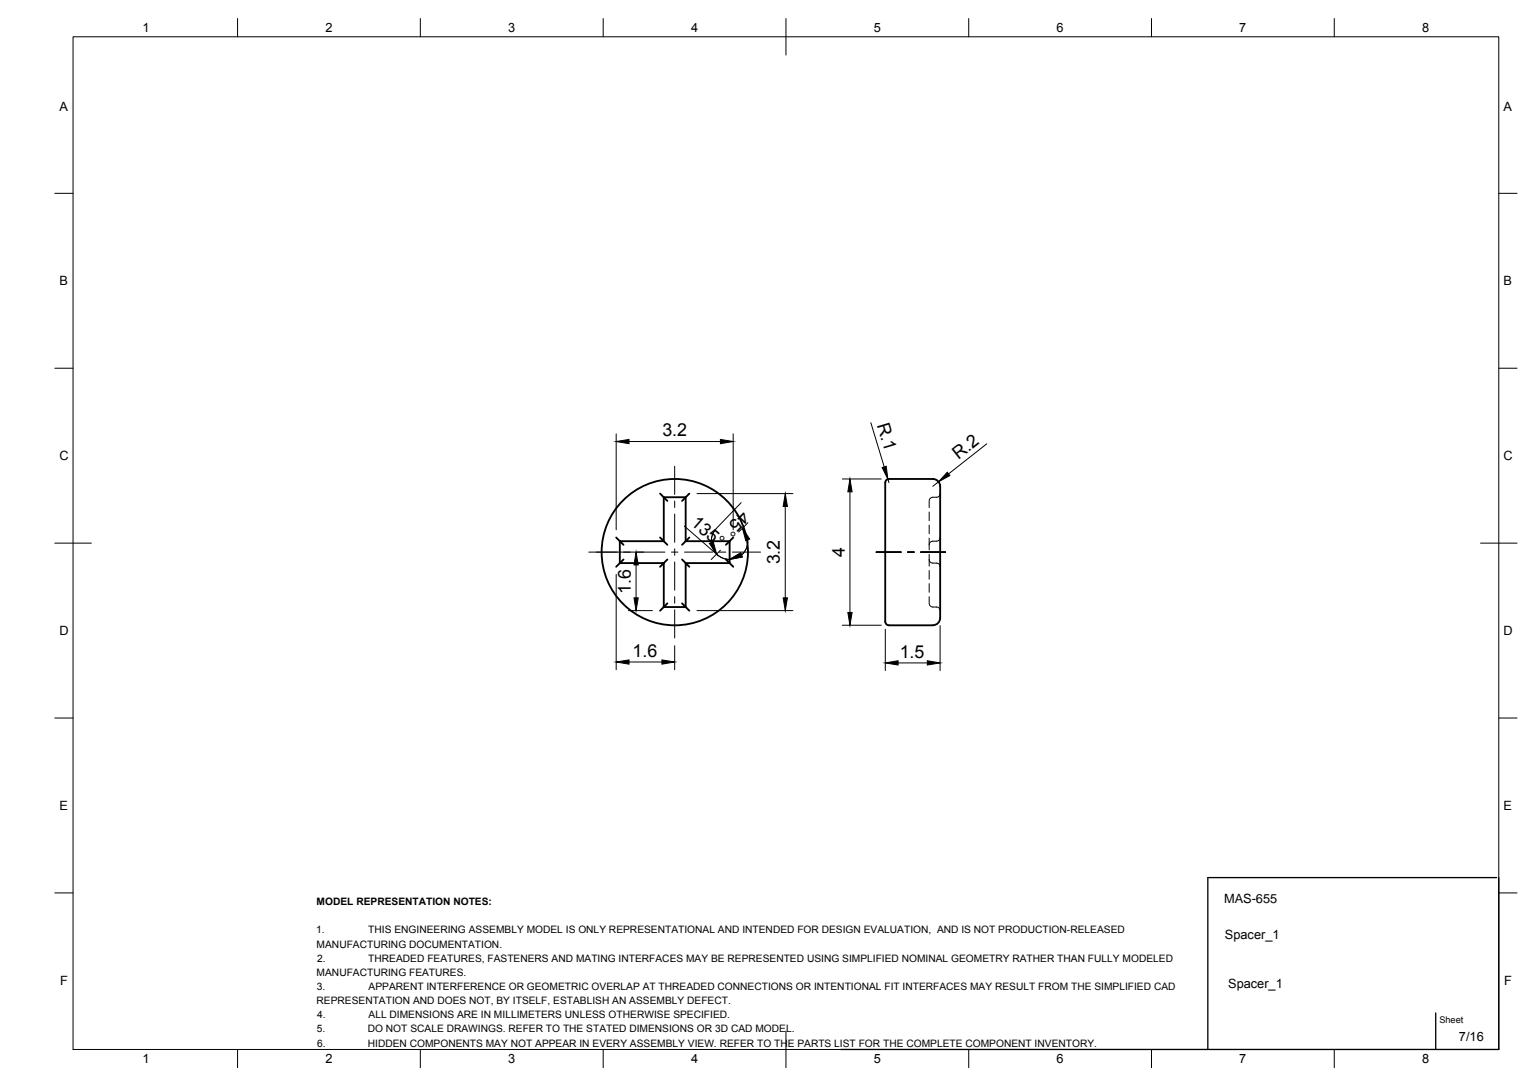
ISO-10303-21;
HEADER;
FILE_DESCRIPTION((''),'2;1');
FILE_NAME('Spacer_1.step','2026-10-09T11:34:15-07:00',(''),(''),'','','');
FILE_SCHEMA (('AUTOMOTIVE_DESIGN { 1 0 10303 214 3 1 1 }'));
ENDSEC;
DATA;
#10=MECHANICAL_DESIGN_GEOMETRIC_PRESENTATION_REPRESENTATION('',(#639),#117170);
#317=ELLIPSE('',#52230,0.141421356237297,0.1) ;
#318=ELLIPSE('',#52231,0.141421356237322,0.1) ;
#319=ELLIPSE('',#52233,0.141421356237322,0.1) ;
#320=ELLIPSE('',#52235,0.141421356237297,0.1) ;
#321=ELLIPSE('',#52237,0.141421356237322,0.1) ;
#322=ELLIPSE('',#52239,0.141421356237297,0.1) ;
#323=ELLIPSE('',#52241,0.141421356237297,0.1) ;
#324=ELLIPSE('',#52242,0.141421356237297,0.1) ;
#325=ELLIPSE('',#52244,0.141421356237322,0.1) ;
#326=ELLIPSE('',#52247,0.141421356237297,0.1) ;
#327=ELLIPSE('',#52249,0.141421356237322,0.1) ;
#328=ELLIPSE('',#52251,0.141421356237297,0.1) ;
#329=ELLIPSE('',#52262,0.141421356237272,0.1) ;
#330=ELLIPSE('',#52263,0.141421356237347,0.1) ;
#331=ELLIPSE('',#52265,0.141421356237347,0.1) ;
#332=ELLIPSE('',#52267,0.141421356237272,0.1) ;
#333=ELLIPSE('',#52269,0.141421356237297,0.1) ;
#334=ELLIPSE('',#52271,0.141421356237322,0.1) ;
#335=ELLIPSE('',#52273,0.141421356237347,0.1) ;
#336=ELLIPSE('',#52275,0.141421356237272,0.1) ;
#337=ELLIPSE('',#52277,0.141421356237347,0.1) ;
#338=ELLIPSE('',#52279,0.141421356237272,0.1) ;
#339=ELLIPSE('',#52281,0.141421356237297,0.1) ;
#340=ELLIPSE('',#52283,0.141421356237322,0.1) ;
#597=SHAPE_REPRESENTATION_RELATIONSHIP('SRR','None',#117252,#618) ;
#618=ADVANCED_BREP_SHAPE_REPRESENTATION('',(#660),#117160) ;
#639=STYLED_ITEM('',(#117355),#660) ;
#660=MANIFOLD_SOLID_BREP('Body1',#49068) ;
#734=FACE_BOUND('',#15393,.T.) ;
#2507=PLANE('',#52228) ;
#2508=PLANE('',#52253) ;
#2509=PLANE('',#52254) ;
#2510=PLANE('',#52255) ;
#2511=PLANE('',#52256) ;
#2512=PLANE('',#52257) ;
#2513=PLANE('',#52258) ;
#2514=PLANE('',#52259) ;
#2515=PLANE('',#52285) ;
#2516=PLANE('',#52286) ;
#2517=PLANE('',#52287) ;
#2518=PLANE('',#52288) ;
#2519=PLANE('',#52291) ;
#2520=PLANE('',#52292) ;
#2521=PLANE('',#52293) ;
#4366=LINE('',#88213,#7580) ;
#4367=LINE('',#88221,#7581) ;
#4368=LINE('',#88225,#7582) ;
#4369=LINE('',#88229,#7583) ;
#4370=LINE('',#88232,#7584) ;
#4371=LINE('',#88235,#7585) ;
#4372=LINE('',#88238,#7586) ;
#4373=LINE('',#88241,#7587) ;
#4374=LINE('',#88244,#7588) ;
#4375=LINE('',#88247,#7589) ;
#4376=LINE('',#88250,#7590) ;
#4377=LINE('',#88254,#7591) ;
#4378=LINE('',#88258,#7592) ;
#4379=LINE('',#88262,#7593) ;
#4380=LINE('',#88264,#7594) ;
#4381=LINE('',#88267,#7595) ;
#4382=LINE('',#88268,#7596) ;
#4383=LINE('',#88271,#7597) ;
#4384=LINE('',#88273,#7598) ;
#4385=LINE('',#88277,#7599) ;
#4386=LINE('',#88279,#7600) ;
#4387=LINE('',#88283,#7601) ;
#4388=LINE('',#88285,#7602) ;
#4389=LINE('',#88288,#7603) ;
#4390=LINE('',#88289,#7604) ;
#4391=LINE('',#88292,#7605) ;
#4392=LINE('',#88294,#7606) ;
#4393=LINE('',#88295,#7607) ;
#4394=LINE('',#88298,#7608) ;
#4395=LINE('',#88299,#7609) ;
#4396=LINE('',#88302,#7610) ;
#4397=LINE('',#88303,#7611) ;
#4398=LINE('',#88306,#7612) ;
#4399=LINE('',#88307,#7613) ;
#4400=LINE('',#88310,#7614) ;
#4401=LINE('',#88311,#7615) ;
#4402=LINE('',#88314,#7616) ;
#4403=LINE('',#88315,#7617) ;
#4404=LINE('',#88322,#7618) ;
#4405=LINE('',#88326,#7619) ;
#4406=LINE('',#88330,#7620) ;
#4407=LINE('',#88333,#7621) ;
#4408=LINE('',#88336,#7622) ;
#4409=LINE('',#88339,#7623) ;
#4410=LINE('',#88342,#7624) ;
#4411=LINE('',#88344,#7625) ;
#4412=LINE('',#88347,#7626) ;
#4413=LINE('',#88351,#7627) ;
#4414=LINE('',#88355,#7628) ;
#4415=LINE('',#88359,#7629) ;
#4416=LINE('',#88363,#7630) ;
#4417=LINE('',#88367,#7631) ;
#4418=LINE('',#88371,#7632) ;
#4419=LINE('',#88373,#7633) ;
#4420=LINE('',#88376,#7634) ;
#4421=LINE('',#88377,#7635) ;
#4422=LINE('',#88379,#7636) ;
#4423=LINE('',#88381,#7637) ;
#4424=LINE('',#88383,#7638) ;
#4425=LINE('',#88388,#7639) ;
#4426=LINE('',#88390,#7640) ;
#7580=VECTOR('',#62263,2.) ;
#7581=VECTOR('',#62272,10.) ;
#7582=VECTOR('',#62275,10.) ;
#7583=VECTOR('',#62280,10.) ;
#7584=VECTOR('',#62283,10.) ;
#7585=VECTOR('',#62286,10.) ;
#7586=VECTOR('',#62289,10.) ;
#7587=VECTOR('',#62292,10.) ;
#7588=VECTOR('',#62295,10.) ;
#7589=VECTOR('',#62298,10.) ;
#7590=VECTOR('',#62301,10.) ;
#7591=VECTOR('',#62304,10.) ;
#7592=VECTOR('',#62307,10.) ;
#7593=VECTOR('',#62312,10.) ;
#7594=VECTOR('',#62313,10.) ;
#7595=VECTOR('',#62318,10.) ;
#7596=VECTOR('',#62319,10.) ;
#7597=VECTOR('',#62322,10.) ;
#7598=VECTOR('',#62323,10.) ;
#7599=VECTOR('',#62328,10.) ;
#7600=VECTOR('',#62329,10.) ;
#7601=VECTOR('',#62334,10.) ;
#7602=VECTOR('',#62335,10.) ;
#7603=VECTOR('',#62340,10.) ;
#7604=VECTOR('',#62341,10.) ;
#7605=VECTOR('',#62344,10.) ;
#7606=VECTOR('',#62345,10.) ;
#7607=VECTOR('',#62346,10.) ;
#7608=VECTOR('',#62349,10.) ;
#7609=VECTOR('',#62350,10.) ;
#7610=VECTOR('',#62353,10.) ;
#7611=VECTOR('',#62354,10.) ;
#7612=VECTOR('',#62357,10.) ;
#7613=VECTOR('',#62358,10.) ;
#7614=VECTOR('',#62361,10.) ;
#7615=VECTOR('',#62362,10.) ;
#7616=VECTOR('',#62365,10.) ;
#7617=VECTOR('',#62366,10.) ;
#7618=VECTOR('',#62373,10.) ;
#7619=VECTOR('',#62376,10.) ;
#7620=VECTOR('',#62381,10.) ;
#7621=VECTOR('',#62384,10.) ;
#7622=VECTOR('',#62387,10.) ;
#7623=VECTOR('',#62390,10.) ;
#7624=VECTOR('',#62393,10.) ;
#7625=VECTOR('',#62396,10.) ;
#7626=VECTOR('',#62399,10.) ;
#7627=VECTOR('',#62404,10.) ;
#7628=VECTOR('',#62409,10.) ;
#7629=VECTOR('',#62414,10.) ;
#7630=VECTOR('',#62419,10.) ;
#7631=VECTOR('',#62424,10.) ;
#7632=VECTOR('',#62429,10.) ;
#7633=VECTOR('',#62430,10.) ;
#7634=VECTOR('',#62435,10.) ;
#7635=VECTOR('',#62436,10.) ;
#7636=VECTOR('',#62439,10.) ;
#7637=VECTOR('',#62442,10.) ;
#7638=VECTOR('',#62445,10.) ;
#7639=VECTOR('',#62454,10.) ;
#7640=VECTOR('',#62457,10.) ;
#10040=CYLINDRICAL_SURFACE('',#52225,2.) ;
#10041=CYLINDRICAL_SURFACE('',#52229,0.1) ;
#10042=CYLINDRICAL_SURFACE('',#52232,0.1) ;
#10043=CYLINDRICAL_SURFACE('',#52234,0.1) ;
#10044=CYLINDRICAL_SURFACE('',#52236,0.1) ;
#10045=CYLINDRICAL_SURFACE('',#52238,0.1) ;
#10046=CYLINDRICAL_SURFACE('',#52240,0.1) ;
#10047=CYLINDRICAL_SURFACE('',#52243,0.1) ;
#10048=CYLINDRICAL_SURFACE('',#52245,0.1) ;
#10049=CYLINDRICAL_SURFACE('',#52246,0.1) ;
#10050=CYLINDRICAL_SURFACE('',#52248,0.1) ;
#10051=CYLINDRICAL_SURFACE('',#52250,0.1) ;
#10052=CYLINDRICAL_SURFACE('',#52252,0.1) ;
#10053=CYLINDRICAL_SURFACE('',#52261,0.1) ;
#10054=CYLINDRICAL_SURFACE('',#52264,0.1) ;
#10055=CYLINDRICAL_SURFACE('',#52266,0.1) ;
#10056=CYLINDRICAL_SURFACE('',#52268,0.1) ;
#10057=CYLINDRICAL_SURFACE('',#52270,0.1) ;
#10058=CYLINDRICAL_SURFACE('',#52272,0.1) ;
#10059=CYLINDRICAL_SURFACE('',#52274,0.1) ;
#10060=CYLINDRICAL_SURFACE('',#52276,0.1) ;
#10061=CYLINDRICAL_SURFACE('',#52278,0.1) ;
#10062=CYLINDRICAL_SURFACE('',#52280,0.1) ;
#10063=CYLINDRICAL_SURFACE('',#52282,0.1) ;
#10064=CYLINDRICAL_SURFACE('',#52284,0.1) ;
#12215=FACE_OUTER_BOUND('',#15371,.T.) ;
#12216=FACE_OUTER_BOUND('',#15372,.T.) ;
#12217=FACE_OUTER_BOUND('',#15373,.T.) ;
#12218=FACE_OUTER_BOUND('',#15374,.T.) ;
#12219=FACE_OUTER_BOUND('',#15375,.T.) ;
#12220=FACE_OUTER_BOUND('',#15376,.T.) ;
#12221=FACE_OUTER_BOUND('',#15377,.T.) ;
#12222=FACE_OUTER_BOUND('',#15378,.T.) ;
#12223=FACE_OUTER_BOUND('',#15379,.T.) ;
#12224=FACE_OUTER_BOUND('',#15380,.T.) ;
#12225=FACE_OUTER_BOUND('',#15381,.T.) ;
#12226=FACE_OUTER_BOUND('',#15382,.T.) ;
#12227=FACE_OUTER_BOUND('',#15383,.T.) ;
#12228=FACE_OUTER_BOUND('',#15384,.T.) ;
#12229=FACE_OUTER_BOUND('',#15385,.T.) ;
#12230=FACE_OUTER_BOUND('',#15386,.T.) ;
#12231=FACE_OUTER_BOUND('',#15387,.T.) ;
#12232=FACE_OUTER_BOUND('',#15388,.T.) ;
#12233=FACE_OUTER_BOUND('',#15389,.T.) ;
#12234=FACE_OUTER_BOUND('',#15390,.T.) ;
#12235=FACE_OUTER_BOUND('',#15391,.T.) ;
#12236=FACE_OUTER_BOUND('',#15392,.T.) ;
#12237=FACE_OUTER_BOUND('',#15394,.T.) ;
#12238=FACE_OUTER_BOUND('',#15395,.T.) ;
#12239=FACE_OUTER_BOUND('',#15396,.T.) ;
#12240=FACE_OUTER_BOUND('',#15397,.T.) ;
#12241=FACE_OUTER_BOUND('',#15398,.T.) ;
#12242=FACE_OUTER_BOUND('',#15399,.T.) ;
#12243=FACE_OUTER_BOUND('',#15400,.T.) ;
#12244=FACE_OUTER_BOUND('',#15401,.T.) ;
#12245=FACE_OUTER_BOUND('',#15402,.T.) ;
#12246=FACE_OUTER_BOUND('',#15403,.T.) ;
#12247=FACE_OUTER_BOUND('',#15404,.T.) ;
#12248=FACE_OUTER_BOUND('',#15405,.T.) ;
#12249=FACE_OUTER_BOUND('',#15406,.T.) ;
#12250=FACE_OUTER_BOUND('',#15407,.T.) ;
#12251=FACE_OUTER_BOUND('',#15408,.T.) ;
#12252=FACE_OUTER_BOUND('',#15409,.T.) ;
#12253=FACE_OUTER_BOUND('',#15410,.T.) ;
#12254=FACE_OUTER_BOUND('',#15411,.T.) ;
#12255=FACE_OUTER_BOUND('',#15412,.T.) ;
#12256=FACE_OUTER_BOUND('',#15413,.T.) ;
#15371=EDGE_LOOP('',(#37742,#37743,#37744,#37745,#37746)) ;
#15372=EDGE_LOOP('',(#37747,#37748,#37749,#37750,#37751,#37752)) ;
#15373=EDGE_LOOP('',(#37753)) ;
#15374=EDGE_LOOP('',(#37754,#37755,#37756,#37757)) ;
#15375=EDGE_LOOP('',(#37758,#37759,#37760,#37761)) ;
#15376=EDGE_LOOP('',(#37762,#37763,#37764,#37765)) ;
#15377=EDGE_LOOP('',(#37766,#37767,#37768,#37769)) ;
#15378=EDGE_LOOP('',(#37770,#37771,#37772,#37773)) ;
#15379=EDGE_LOOP('',(#37774,#37775,#37776,#37777)) ;
#15380=EDGE_LOOP('',(#37778,#37779,#37780,#37781)) ;
#15381=EDGE_LOOP('',(#37782,#37783,#37784,#37785)) ;
#15382=EDGE_LOOP('',(#37786,#37787,#37788,#37789)) ;
#15383=EDGE_LOOP('',(#37790,#37791,#37792,#37793)) ;
#15384=EDGE_LOOP('',(#37794,#37795,#37796,#37797)) ;
#15385=EDGE_LOOP('',(#37798,#37799,#37800,#37801)) ;
#15386=EDGE_LOOP('',(#37802,#37803,#37804,#37805)) ;
#15387=EDGE_LOOP('',(#37806,#37807,#37808,#37809)) ;
#15388=EDGE_LOOP('',(#37810,#37811,#37812,#37813)) ;
#15389=EDGE_LOOP('',(#37814,#37815,#37816,#37817)) ;
#15390=EDGE_LOOP('',(#37818,#37819,#37820,#37821)) ;
#15391=EDGE_LOOP('',(#37822,#37823,#37824,#37825)) ;
#15392=EDGE_LOOP('',(#37826)) ;
#15393=EDGE_LOOP('',(#37827,#37828,#37829,#37830,#37831,#37832,#37833,#37834,
#37835,#37836,#37837,#37838)) ;
#15394=EDGE_LOOP('',(#37839,#37840,#37841,#37842)) ;
#15395=EDGE_LOOP('',(#37843,#37844,#37845,#37846)) ;
#15396=EDGE_LOOP('',(#37847,#37848,#37849,#37850)) ;
#15397=EDGE_LOOP('',(#37851,#37852,#37853,#37854)) ;
#15398=EDGE_LOOP('',(#37855,#37856,#37857,#37858)) ;
#15399=EDGE_LOOP('',(#37859,#37860,#37861,#37862)) ;
#15400=EDGE_LOOP('',(#37863,#37864,#37865,#37866)) ;
#15401=EDGE_LOOP('',(#37867,#37868,#37869,#37870)) ;
#15402=EDGE_LOOP('',(#37871,#37872,#37873,#37874)) ;
#15403=EDGE_LOOP('',(#37875,#37876,#37877,#37878)) ;
#15404=EDGE_LOOP('',(#37879,#37880,#37881,#37882)) ;
#15405=EDGE_LOOP('',(#37883,#37884,#37885,#37886)) ;
#15406=EDGE_LOOP('',(#37887,#37888,#37889,#37890)) ;
#15407=EDGE_LOOP('',(#37891,#37892,#37893,#37894)) ;
#15408=EDGE_LOOP('',(#37895,#37896,#37897,#37898)) ;
#15409=EDGE_LOOP('',(#37899,#37900,#37901,#37902,#37903,#37904,#37905,#37906,
#37907,#37908,#37909,#37910)) ;
#15410=EDGE_LOOP('',(#37911,#37912,#37913,#37914,#37915)) ;
#15411=EDGE_LOOP('',(#37916,#37917,#37918,#37919)) ;
#15412=EDGE_LOOP('',(#37920,#37921,#37922,#37923)) ;
#15413=EDGE_LOOP('',(#37924,#37925,#37926,#37927)) ;
#18485=CIRCLE('',#52221,1.9) ;
#18486=CIRCLE('',#52222,0.1) ;
#18487=CIRCLE('',#52223,2.) ;
#18488=CIRCLE('',#52224,2.) ;
#18489=CIRCLE('',#52226,2.) ;
#18490=CIRCLE('',#52227,2.) ;
#18491=CIRCLE('',#52260,1.8) ;
#18492=CIRCLE('',#52290,0.2) ;
#21507=VERTEX_POINT('',#88204) ;
#21508=VERTEX_POINT('',#88206) ;
#21509=VERTEX_POINT('',#88208) ;
#21510=VERTEX_POINT('',#88212) ;
#21511=VERTEX_POINT('',#88214) ;
#21512=VERTEX_POINT('',#88219) ;
#21513=VERTEX_POINT('',#88220) ;
#21514=VERTEX_POINT('',#88222) ;
#21515=VERTEX_POINT('',#88224) ;
#21516=VERTEX_POINT('',#88228) ;
#21517=VERTEX_POINT('',#88230) ;
#21518=VERTEX_POINT('',#88234) ;
#21519=VERTEX_POINT('',#88236) ;
#21520=VERTEX_POINT('',#88240) ;
#21521=VERTEX_POINT('',#88242) ;
#21522=VERTEX_POINT('',#88246) ;
#21523=VERTEX_POINT('',#88248) ;
#21524=VERTEX_POINT('',#88252) ;
#21525=VERTEX_POINT('',#88253) ;
#21526=VERTEX_POINT('',#88255) ;
#21527=VERTEX_POINT('',#88257) ;
#21528=VERTEX_POINT('',#88261) ;
#21529=VERTEX_POINT('',#88263) ;
#21530=VERTEX_POINT('',#88270) ;
#21531=VERTEX_POINT('',#88272) ;
#21532=VERTEX_POINT('',#88276) ;
#21533=VERTEX_POINT('',#88278) ;
#21534=VERTEX_POINT('',#88282) ;
#21535=VERTEX_POINT('',#88284) ;
#21536=VERTEX_POINT('',#88291) ;
#21537=VERTEX_POINT('',#88293) ;
#21538=VERTEX_POINT('',#88297) ;
#21539=VERTEX_POINT('',#88301) ;
#21540=VERTEX_POINT('',#88305) ;
#21541=VERTEX_POINT('',#88309) ;
#21542=VERTEX_POINT('',#88313) ;
#21543=VERTEX_POINT('',#88317) ;
#21544=VERTEX_POINT('',#88320) ;
#21545=VERTEX_POINT('',#88321) ;
#21546=VERTEX_POINT('',#88323) ;
#21547=VERTEX_POINT('',#88325) ;
#21548=VERTEX_POINT('',#88329) ;
#21549=VERTEX_POINT('',#88331) ;
#21550=VERTEX_POINT('',#88335) ;
#21551=VERTEX_POINT('',#88337) ;
#21552=VERTEX_POINT('',#88341) ;
#21553=VERTEX_POINT('',#88346) ;
#21554=VERTEX_POINT('',#88350) ;
#21555=VERTEX_POINT('',#88354) ;
#21556=VERTEX_POINT('',#88358) ;
#21557=VERTEX_POINT('',#88362) ;
#21558=VERTEX_POINT('',#88366) ;
#21559=VERTEX_POINT('',#88370) ;
#21560=VERTEX_POINT('',#88372) ;
#27149=EDGE_CURVE('',#21507,#21507,#18485,.T.) ;
#27150=EDGE_CURVE('',#21507,#21508,#18486,.T.) ;
#27151=EDGE_CURVE('',#21508,#21509,#18487,.T.) ;
#27152=EDGE_CURVE('',#21509,#21508,#18488,.T.) ;
#27153=EDGE_CURVE('',#21509,#21510,#4366,.T.) ;
#27154=EDGE_CURVE('',#21511,#21510,#18489,.T.) ;
#27155=EDGE_CURVE('',#21510,#21511,#18490,.T.) ;
#27156=EDGE_CURVE('',#21512,#21513,#4367,.T.) ;
#27157=EDGE_CURVE('',#21513,#21514,#317,.T.) ;
#27158=EDGE_CURVE('',#21514,#21515,#4368,.T.) ;
#27159=EDGE_CURVE('',#21512,#21515,#318,.T.) ;
#27160=EDGE_CURVE('',#21513,#21516,#4369,.T.) ;
#27161=EDGE_CURVE('',#21516,#21517,#319,.T.) ;
#27162=EDGE_CURVE('',#21517,#21514,#4370,.T.) ;
#27163=EDGE_CURVE('',#21516,#21518,#4371,.T.) ;
#27164=EDGE_CURVE('',#21518,#21519,#320,.T.) ;
#27165=EDGE_CURVE('',#21519,#21517,#4372,.T.) ;
#27166=EDGE_CURVE('',#21518,#21520,#4373,.T.) ;
#27167=EDGE_CURVE('',#21520,#21521,#321,.T.) ;
#27168=EDGE_CURVE('',#21521,#21519,#4374,.T.) ;
#27169=EDGE_CURVE('',#21520,#21522,#4375,.T.) ;
#27170=EDGE_CURVE('',#21522,#21523,#322,.T.) ;
#27171=EDGE_CURVE('',#21523,#21521,#4376,.T.) ;
#27172=EDGE_CURVE('',#21524,#21525,#4377,.T.) ;
#27173=EDGE_CURVE('',#21525,#21526,#323,.T.) ;
#27174=EDGE_CURVE('',#21526,#21527,#4378,.T.) ;
#27175=EDGE_CURVE('',#21527,#21524,#324,.T.) ;
#27176=EDGE_CURVE('',#21528,#21526,#4379,.T.) ;
#27177=EDGE_CURVE('',#21525,#21529,#4380,.T.) ;
#27178=EDGE_CURVE('',#21529,#21528,#325,.T.) ;
#27179=EDGE_CURVE('',#21522,#21524,#4381,.T.) ;
#27180=EDGE_CURVE('',#21527,#21523,#4382,.T.) ;
#27181=EDGE_CURVE('',#21530,#21528,#4383,.T.) ;
#27182=EDGE_CURVE('',#21529,#21531,#4384,.T.) ;
#27183=EDGE_CURVE('',#21531,#21530,#326,.T.) ;
#27184=EDGE_CURVE('',#21532,#21530,#4385,.T.) ;
#27185=EDGE_CURVE('',#21531,#21533,#4386,.T.) ;
#27186=EDGE_CURVE('',#21533,#21532,#327,.T.) ;
#27187=EDGE_CURVE('',#21534,#21532,#4387,.T.) ;
#27188=EDGE_CURVE('',#21533,#21535,#4388,.T.) ;
#27189=EDGE_CURVE('',#21535,#21534,#328,.T.) ;
#27190=EDGE_CURVE('',#21515,#21534,#4389,.T.) ;
#27191=EDGE_CURVE('',#21535,#21512,#4390,.T.) ;
#27192=EDGE_CURVE('',#21517,#21536,#4391,.T.) ;
#27193=EDGE_CURVE('',#21537,#21536,#4392,.T.) ;
#27194=EDGE_CURVE('',#21514,#21537,#4393,.T.) ;
#27195=EDGE_CURVE('',#21519,#21538,#4394,.T.) ;
#27196=EDGE_CURVE('',#21536,#21538,#4395,.T.) ;
#27197=EDGE_CURVE('',#21521,#21539,#4396,.T.) ;
#27198=EDGE_CURVE('',#21538,#21539,#4397,.T.) ;
#27199=EDGE_CURVE('',#21523,#21540,#4398,.T.) ;
#27200=EDGE_CURVE('',#21539,#21540,#4399,.T.) ;
#27201=EDGE_CURVE('',#21527,#21541,#4400,.T.) ;
#27202=EDGE_CURVE('',#21540,#21541,#4401,.T.) ;
#27203=EDGE_CURVE('',#21526,#21542,#4402,.T.) ;
#27204=EDGE_CURVE('',#21541,#21542,#4403,.T.) ;
#27205=EDGE_CURVE('',#21543,#21543,#18491,.T.) ;
#27206=EDGE_CURVE('',#21544,#21545,#4404,.T.) ;
#27207=EDGE_CURVE('',#21545,#21546,#329,.T.) ;
#27208=EDGE_CURVE('',#21546,#21547,#4405,.T.) ;
#27209=EDGE_CURVE('',#21544,#21547,#330,.T.) ;
#27210=EDGE_CURVE('',#21545,#21548,#4406,.T.) ;
#27211=EDGE_CURVE('',#21548,#21549,#331,.T.) ;
#27212=EDGE_CURVE('',#21549,#21546,#4407,.T.) ;
#27213=EDGE_CURVE('',#21548,#21550,#4408,.T.) ;
#27214=EDGE_CURVE('',#21550,#21551,#332,.T.) ;
#27215=EDGE_CURVE('',#21551,#21549,#4409,.T.) ;
#27216=EDGE_CURVE('',#21550,#21552,#4410,.T.) ;
#27217=EDGE_CURVE('',#21552,#21542,#333,.T.) ;
#27218=EDGE_CURVE('',#21542,#21551,#4411,.T.) ;
#27219=EDGE_CURVE('',#21552,#21553,#4412,.T.) ;
#27220=EDGE_CURVE('',#21553,#21541,#334,.T.) ;
#27221=EDGE_CURVE('',#21553,#21554,#4413,.T.) ;
#27222=EDGE_CURVE('',#21554,#21540,#335,.T.) ;
#27223=EDGE_CURVE('',#21554,#21555,#4414,.T.) ;
#27224=EDGE_CURVE('',#21555,#21539,#336,.T.) ;
#27225=EDGE_CURVE('',#21555,#21556,#4415,.T.) ;
#27226=EDGE_CURVE('',#21556,#21538,#337,.T.) ;
#27227=EDGE_CURVE('',#21556,#21557,#4416,.T.) ;
#27228=EDGE_CURVE('',#21557,#21536,#338,.T.) ;
#27229=EDGE_CURVE('',#21557,#21558,#4417,.T.) ;
#27230=EDGE_CURVE('',#21558,#21537,#339,.T.) ;
#27231=EDGE_CURVE('',#21559,#21537,#4418,.T.) ;
#27232=EDGE_CURVE('',#21558,#21560,#4419,.T.) ;
#27233=EDGE_CURVE('',#21560,#21559,#340,.T.) ;
#27234=EDGE_CURVE('',#21547,#21559,#4420,.T.) ;
#27235=EDGE_CURVE('',#21560,#21544,#4421,.T.) ;
#27236=EDGE_CURVE('',#21515,#21559,#4422,.T.) ;
#27237=EDGE_CURVE('',#21534,#21547,#4423,.T.) ;
#27238=EDGE_CURVE('',#21532,#21546,#4424,.T.) ;
#27239=EDGE_CURVE('',#21511,#21543,#18492,.T.) ;
#27240=EDGE_CURVE('',#21530,#21549,#4425,.T.) ;
#27241=EDGE_CURVE('',#21528,#21551,#4426,.T.) ;
#37742=ORIENTED_EDGE('',*,*,#27149,.T.) ;
#37743=ORIENTED_EDGE('',*,*,#27150,.T.) ;
#37744=ORIENTED_EDGE('',*,*,#27151,.T.) ;
#37745=ORIENTED_EDGE('',*,*,#27152,.T.) ;
#37746=ORIENTED_EDGE('',*,*,#27150,.F.) ;
#37747=ORIENTED_EDGE('',*,*,#27152,.F.) ;
#37748=ORIENTED_EDGE('',*,*,#27153,.T.) ;
#37749=ORIENTED_EDGE('',*,*,#27154,.F.) ;
#37750=ORIENTED_EDGE('',*,*,#27155,.F.) ;
#37751=ORIENTED_EDGE('',*,*,#27153,.F.) ;
#37752=ORIENTED_EDGE('',*,*,#27151,.F.) ;
#37753=ORIENTED_EDGE('',*,*,#27149,.F.) ;
#37754=ORIENTED_EDGE('',*,*,#27156,.T.) ;
#37755=ORIENTED_EDGE('',*,*,#27157,.T.) ;
#37756=ORIENTED_EDGE('',*,*,#27158,.T.) ;
#37757=ORIENTED_EDGE('',*,*,#27159,.F.) ;
#37758=ORIENTED_EDGE('',*,*,#27160,.T.) ;
#37759=ORIENTED_EDGE('',*,*,#27161,.T.) ;
#37760=ORIENTED_EDGE('',*,*,#27162,.T.) ;
#37761=ORIENTED_EDGE('',*,*,#27157,.F.) ;
#37762=ORIENTED_EDGE('',*,*,#27163,.T.) ;
#37763=ORIENTED_EDGE('',*,*,#27164,.T.) ;
#37764=ORIENTED_EDGE('',*,*,#27165,.T.) ;
#37765=ORIENTED_EDGE('',*,*,#27161,.F.) ;
#37766=ORIENTED_EDGE('',*,*,#27166,.T.) ;
#37767=ORIENTED_EDGE('',*,*,#27167,.T.) ;
#37768=ORIENTED_EDGE('',*,*,#27168,.T.) ;
#37769=ORIENTED_EDGE('',*,*,#27164,.F.) ;
#37770=ORIENTED_EDGE('',*,*,#27169,.T.) ;
#37771=ORIENTED_EDGE('',*,*,#27170,.T.) ;
#37772=ORIENTED_EDGE('',*,*,#27171,.T.) ;
#37773=ORIENTED_EDGE('',*,*,#27167,.F.) ;
#37774=ORIENTED_EDGE('',*,*,#27172,.T.) ;
#37775=ORIENTED_EDGE('',*,*,#27173,.T.) ;
#37776=ORIENTED_EDGE('',*,*,#27174,.T.) ;
#37777=ORIENTED_EDGE('',*,*,#27175,.T.) ;
#37778=ORIENTED_EDGE('',*,*,#27176,.T.) ;
#37779=ORIENTED_EDGE('',*,*,#27173,.F.) ;
#37780=ORIENTED_EDGE('',*,*,#27177,.T.) ;
#37781=ORIENTED_EDGE('',*,*,#27178,.T.) ;
#37782=ORIENTED_EDGE('',*,*,#27179,.T.) ;
#37783=ORIENTED_EDGE('',*,*,#27175,.F.) ;
#37784=ORIENTED_EDGE('',*,*,#27180,.T.) ;
#37785=ORIENTED_EDGE('',*,*,#27170,.F.) ;
#37786=ORIENTED_EDGE('',*,*,#27181,.T.) ;
#37787=ORIENTED_EDGE('',*,*,#27178,.F.) ;
#37788=ORIENTED_EDGE('',*,*,#27182,.T.) ;
#37789=ORIENTED_EDGE('',*,*,#27183,.T.) ;
#37790=ORIENTED_EDGE('',*,*,#27184,.T.) ;
#37791=ORIENTED_EDGE('',*,*,#27183,.F.) ;
#37792=ORIENTED_EDGE('',*,*,#27185,.T.) ;
#37793=ORIENTED_EDGE('',*,*,#27186,.T.) ;
#37794=ORIENTED_EDGE('',*,*,#27187,.T.) ;
#37795=ORIENTED_EDGE('',*,*,#27186,.F.) ;
#37796=ORIENTED_EDGE('',*,*,#27188,.T.) ;
#37797=ORIENTED_EDGE('',*,*,#27189,.T.) ;
#37798=ORIENTED_EDGE('',*,*,#27190,.T.) ;
#37799=ORIENTED_EDGE('',*,*,#27189,.F.) ;
#37800=ORIENTED_EDGE('',*,*,#27191,.T.) ;
#37801=ORIENTED_EDGE('',*,*,#27159,.T.) ;
#37802=ORIENTED_EDGE('',*,*,#27162,.F.) ;
#37803=ORIENTED_EDGE('',*,*,#27192,.T.) ;
#37804=ORIENTED_EDGE('',*,*,#27193,.F.) ;
#37805=ORIENTED_EDGE('',*,*,#27194,.F.) ;
#37806=ORIENTED_EDGE('',*,*,#27165,.F.) ;
#37807=ORIENTED_EDGE('',*,*,#27195,.T.) ;
#37808=ORIENTED_EDGE('',*,*,#27196,.F.) ;
#37809=ORIENTED_EDGE('',*,*,#27192,.F.) ;
#37810=ORIENTED_EDGE('',*,*,#27168,.F.) ;
#37811=ORIENTED_EDGE('',*,*,#27197,.T.) ;
#37812=ORIENTED_EDGE('',*,*,#27198,.F.) ;
#37813=ORIENTED_EDGE('',*,*,#27195,.F.) ;
#37814=ORIENTED_EDGE('',*,*,#27171,.F.) ;
#37815=ORIENTED_EDGE('',*,*,#27199,.T.) ;
#37816=ORIENTED_EDGE('',*,*,#27200,.F.) ;
#37817=ORIENTED_EDGE('',*,*,#27197,.F.) ;
#37818=ORIENTED_EDGE('',*,*,#27180,.F.) ;
#37819=ORIENTED_EDGE('',*,*,#27201,.T.) ;
#37820=ORIENTED_EDGE('',*,*,#27202,.F.) ;
#37821=ORIENTED_EDGE('',*,*,#27199,.F.) ;
#37822=ORIENTED_EDGE('',*,*,#27174,.F.) ;
#37823=ORIENTED_EDGE('',*,*,#27203,.T.) ;
#37824=ORIENTED_EDGE('',*,*,#27204,.F.) ;
#37825=ORIENTED_EDGE('',*,*,#27201,.F.) ;
#37826=ORIENTED_EDGE('',*,*,#27205,.F.) ;
#37827=ORIENTED_EDGE('',*,*,#27172,.F.) ;
#37828=ORIENTED_EDGE('',*,*,#27179,.F.) ;
#37829=ORIENTED_EDGE('',*,*,#27169,.F.) ;
#37830=ORIENTED_EDGE('',*,*,#27166,.F.) ;
#37831=ORIENTED_EDGE('',*,*,#27163,.F.) ;
#37832=ORIENTED_EDGE('',*,*,#27160,.F.) ;
#37833=ORIENTED_EDGE('',*,*,#27156,.F.) ;
#37834=ORIENTED_EDGE('',*,*,#27191,.F.) ;
#37835=ORIENTED_EDGE('',*,*,#27188,.F.) ;
#37836=ORIENTED_EDGE('',*,*,#27185,.F.) ;
#37837=ORIENTED_EDGE('',*,*,#27182,.F.) ;
#37838=ORIENTED_EDGE('',*,*,#27177,.F.) ;
#37839=ORIENTED_EDGE('',*,*,#27206,.T.) ;
#37840=ORIENTED_EDGE('',*,*,#27207,.T.) ;
#37841=ORIENTED_EDGE('',*,*,#27208,.T.) ;
#37842=ORIENTED_EDGE('',*,*,#27209,.F.) ;
#37843=ORIENTED_EDGE('',*,*,#27210,.T.) ;
#37844=ORIENTED_EDGE('',*,*,#27211,.T.) ;
#37845=ORIENTED_EDGE('',*,*,#27212,.T.) ;
#37846=ORIENTED_EDGE('',*,*,#27207,.F.) ;
#37847=ORIENTED_EDGE('',*,*,#27213,.T.) ;
#37848=ORIENTED_EDGE('',*,*,#27214,.T.) ;
#37849=ORIENTED_EDGE('',*,*,#27215,.T.) ;
#37850=ORIENTED_EDGE('',*,*,#27211,.F.) ;
#37851=ORIENTED_EDGE('',*,*,#27216,.T.) ;
#37852=ORIENTED_EDGE('',*,*,#27217,.T.) ;
#37853=ORIENTED_EDGE('',*,*,#27218,.T.) ;
#37854=ORIENTED_EDGE('',*,*,#27214,.F.) ;
#37855=ORIENTED_EDGE('',*,*,#27219,.T.) ;
#37856=ORIENTED_EDGE('',*,*,#27220,.T.) ;
#37857=ORIENTED_EDGE('',*,*,#27204,.T.) ;
#37858=ORIENTED_EDGE('',*,*,#27217,.F.) ;
#37859=ORIENTED_EDGE('',*,*,#27202,.T.) ;
#37860=ORIENTED_EDGE('',*,*,#27220,.F.) ;
#37861=ORIENTED_EDGE('',*,*,#27221,.T.) ;
#37862=ORIENTED_EDGE('',*,*,#27222,.T.) ;
#37863=ORIENTED_EDGE('',*,*,#27200,.T.) ;
#37864=ORIENTED_EDGE('',*,*,#27222,.F.) ;
#37865=ORIENTED_EDGE('',*,*,#27223,.T.) ;
#37866=ORIENTED_EDGE('',*,*,#27224,.T.) ;
#37867=ORIENTED_EDGE('',*,*,#27198,.T.) ;
#37868=ORIENTED_EDGE('',*,*,#27224,.F.) ;
#37869=ORIENTED_EDGE('',*,*,#27225,.T.) ;
#37870=ORIENTED_EDGE('',*,*,#27226,.T.) ;
#37871=ORIENTED_EDGE('',*,*,#27196,.T.) ;
#37872=ORIENTED_EDGE('',*,*,#27226,.F.) ;
#37873=ORIENTED_EDGE('',*,*,#27227,.T.) ;
#37874=ORIENTED_EDGE('',*,*,#27228,.T.) ;
#37875=ORIENTED_EDGE('',*,*,#27193,.T.) ;
#37876=ORIENTED_EDGE('',*,*,#27228,.F.) ;
#37877=ORIENTED_EDGE('',*,*,#27229,.T.) ;
#37878=ORIENTED_EDGE('',*,*,#27230,.T.) ;
#37879=ORIENTED_EDGE('',*,*,#27231,.T.) ;
#37880=ORIENTED_EDGE('',*,*,#27230,.F.) ;
#37881=ORIENTED_EDGE('',*,*,#27232,.T.) ;
#37882=ORIENTED_EDGE('',*,*,#27233,.T.) ;
#37883=ORIENTED_EDGE('',*,*,#27234,.T.) ;
#37884=ORIENTED_EDGE('',*,*,#27233,.F.) ;
#37885=ORIENTED_EDGE('',*,*,#27235,.T.) ;
#37886=ORIENTED_EDGE('',*,*,#27209,.T.) ;
#37887=ORIENTED_EDGE('',*,*,#27158,.F.) ;
#37888=ORIENTED_EDGE('',*,*,#27194,.T.) ;
#37889=ORIENTED_EDGE('',*,*,#27231,.F.) ;
#37890=ORIENTED_EDGE('',*,*,#27236,.F.) ;
#37891=ORIENTED_EDGE('',*,*,#27190,.F.) ;
#37892=ORIENTED_EDGE('',*,*,#27236,.T.) ;
#37893=ORIENTED_EDGE('',*,*,#27234,.F.) ;
#37894=ORIENTED_EDGE('',*,*,#27237,.F.) ;
#37895=ORIENTED_EDGE('',*,*,#27187,.F.) ;
#37896=ORIENTED_EDGE('',*,*,#27237,.T.) ;
#37897=ORIENTED_EDGE('',*,*,#27208,.F.) ;
#37898=ORIENTED_EDGE('',*,*,#27238,.F.) ;
#37899=ORIENTED_EDGE('',*,*,#27206,.F.) ;
#37900=ORIENTED_EDGE('',*,*,#27235,.F.) ;
#37901=ORIENTED_EDGE('',*,*,#27232,.F.) ;
#37902=ORIENTED_EDGE('',*,*,#27229,.F.) ;
#37903=ORIENTED_EDGE('',*,*,#27227,.F.) ;
#37904=ORIENTED_EDGE('',*,*,#27225,.F.) ;
#37905=ORIENTED_EDGE('',*,*,#27223,.F.) ;
#37906=ORIENTED_EDGE('',*,*,#27221,.F.) ;
#37907=ORIENTED_EDGE('',*,*,#27219,.F.) ;
#37908=ORIENTED_EDGE('',*,*,#27216,.F.) ;
#37909=ORIENTED_EDGE('',*,*,#27213,.F.) ;
#37910=ORIENTED_EDGE('',*,*,#27210,.F.) ;
#37911=ORIENTED_EDGE('',*,*,#27154,.T.) ;
#37912=ORIENTED_EDGE('',*,*,#27155,.T.) ;
#37913=ORIENTED_EDGE('',*,*,#27239,.T.) ;
#37914=ORIENTED_EDGE('',*,*,#27205,.T.) ;
#37915=ORIENTED_EDGE('',*,*,#27239,.F.) ;
#37916=ORIENTED_EDGE('',*,*,#27184,.F.) ;
#37917=ORIENTED_EDGE('',*,*,#27238,.T.) ;
#37918=ORIENTED_EDGE('',*,*,#27212,.F.) ;
#37919=ORIENTED_EDGE('',*,*,#27240,.F.) ;
#37920=ORIENTED_EDGE('',*,*,#27181,.F.) ;
#37921=ORIENTED_EDGE('',*,*,#27240,.T.) ;
#37922=ORIENTED_EDGE('',*,*,#27215,.F.) ;
#37923=ORIENTED_EDGE('',*,*,#27241,.F.) ;
#37924=ORIENTED_EDGE('',*,*,#27176,.F.) ;
#37925=ORIENTED_EDGE('',*,*,#27241,.T.) ;
#37926=ORIENTED_EDGE('',*,*,#27218,.F.) ;
#37927=ORIENTED_EDGE('',*,*,#27203,.F.) ;
#45707=TOROIDAL_SURFACE('',#52220,1.9,0.1) ;
#45708=TOROIDAL_SURFACE('',#52289,1.8,0.2) ;
#47433=ADVANCED_FACE('',(#12215),#45707,.T.) ;
#47434=ADVANCED_FACE('',(#12216),#10040,.T.) ;
#47435=ADVANCED_FACE('',(#12217),#2507,.T.) ;
#47436=ADVANCED_FACE('',(#12218),#10041,.T.) ;
#47437=ADVANCED_FACE('',(#12219),#10042,.T.) ;
#47438=ADVANCED_FACE('',(#12220),#10043,.T.) ;
#47439=ADVANCED_FACE('',(#12221),#10044,.T.) ;
#47440=ADVANCED_FACE('',(#12222),#10045,.T.) ;
#47441=ADVANCED_FACE('',(#12223),#10046,.T.) ;
#47442=ADVANCED_FACE('',(#12224),#10047,.T.) ;
#47443=ADVANCED_FACE('',(#12225),#10048,.T.) ;
#47444=ADVANCED_FACE('',(#12226),#10049,.T.) ;
#47445=ADVANCED_FACE('',(#12227),#10050,.T.) ;
#47446=ADVANCED_FACE('',(#12228),#10051,.T.) ;
#47447=ADVANCED_FACE('',(#12229),#10052,.T.) ;
#47448=ADVANCED_FACE('',(#12230),#2508,.F.) ;
#47449=ADVANCED_FACE('',(#12231),#2509,.F.) ;
#47450=ADVANCED_FACE('',(#12232),#2510,.F.) ;
#47451=ADVANCED_FACE('',(#12233),#2511,.F.) ;
#47452=ADVANCED_FACE('',(#12234),#2512,.F.) ;
#47453=ADVANCED_FACE('',(#12235),#2513,.F.) ;
#47454=ADVANCED_FACE('',(#12236,#734),#2514,.F.) ;
#47455=ADVANCED_FACE('',(#12237),#10053,.F.) ;
#47456=ADVANCED_FACE('',(#12238),#10054,.F.) ;
#47457=ADVANCED_FACE('',(#12239),#10055,.F.) ;
#47458=ADVANCED_FACE('',(#12240),#10056,.F.) ;
#47459=ADVANCED_FACE('',(#12241),#10057,.F.) ;
#47460=ADVANCED_FACE('',(#12242),#10058,.F.) ;
#47461=ADVANCED_FACE('',(#12243),#10059,.F.) ;
#47462=ADVANCED_FACE('',(#12244),#10060,.F.) ;
#47463=ADVANCED_FACE('',(#12245),#10061,.F.) ;
#47464=ADVANCED_FACE('',(#12246),#10062,.F.) ;
#47465=ADVANCED_FACE('',(#12247),#10063,.F.) ;
#47466=ADVANCED_FACE('',(#12248),#10064,.F.) ;
#47467=ADVANCED_FACE('',(#12249),#2515,.F.) ;
#47468=ADVANCED_FACE('',(#12250),#2516,.F.) ;
#47469=ADVANCED_FACE('',(#12251),#2517,.F.) ;
#47470=ADVANCED_FACE('',(#12252),#2518,.F.) ;
#47471=ADVANCED_FACE('',(#12253),#45708,.T.) ;
#47472=ADVANCED_FACE('',(#12254),#2519,.F.) ;
#47473=ADVANCED_FACE('',(#12255),#2520,.F.) ;
#47474=ADVANCED_FACE('',(#12256),#2521,.F.) ;
#49068=CLOSED_SHELL('',(#47433,#47434,#47435,#47436,#47437,#47438,#47439,
#47440,#47441,#47442,#47443,#47444,#47445,#47446,#47447,#47448,#47449,#47450,
#47451,#47452,#47453,#47454,#47455,#47456,#47457,#47458,#47459,#47460,#47461,
#47462,#47463,#47464,#47465,#47466,#47467,#47468,#47469,#47470,#47471,#47472,
#47473,#47474)) ;
#52219=AXIS2_PLACEMENT_3D('',#88202,#62249,#62250) ;
#52220=AXIS2_PLACEMENT_3D('',#88203,#62251,#62252) ;
#52221=AXIS2_PLACEMENT_3D('',#88205,#62253,#62254) ;
#52222=AXIS2_PLACEMENT_3D('',#88207,#62255,#62256) ;
#52223=AXIS2_PLACEMENT_3D('',#88209,#62257,#62258) ;
#52224=AXIS2_PLACEMENT_3D('',#88210,#62259,#62260) ;
#52225=AXIS2_PLACEMENT_3D('',#88211,#62261,#62262) ;
#52226=AXIS2_PLACEMENT_3D('',#88215,#62264,#62265) ;
#52227=AXIS2_PLACEMENT_3D('',#88216,#62266,#62267) ;
#52228=AXIS2_PLACEMENT_3D('',#88217,#62268,#62269) ;
#52229=AXIS2_PLACEMENT_3D('',#88218,#62270,#62271) ;
#52230=AXIS2_PLACEMENT_3D('',#88223,#62273,#62274) ;
#52231=AXIS2_PLACEMENT_3D('',#88226,#62276,#62277) ;
#52232=AXIS2_PLACEMENT_3D('',#88227,#62278,#62279) ;
#52233=AXIS2_PLACEMENT_3D('',#88231,#62281,#62282) ;
#52234=AXIS2_PLACEMENT_3D('',#88233,#62284,#62285) ;
#52235=AXIS2_PLACEMENT_3D('',#88237,#62287,#62288) ;
#52236=AXIS2_PLACEMENT_3D('',#88239,#62290,#62291) ;
#52237=AXIS2_PLACEMENT_3D('',#88243,#62293,#62294) ;
#52238=AXIS2_PLACEMENT_3D('',#88245,#62296,#62297) ;
#52239=AXIS2_PLACEMENT_3D('',#88249,#62299,#62300) ;
#52240=AXIS2_PLACEMENT_3D('',#88251,#62302,#62303) ;
#52241=AXIS2_PLACEMENT_3D('',#88256,#62305,#62306) ;
#52242=AXIS2_PLACEMENT_3D('',#88259,#62308,#62309) ;
#52243=AXIS2_PLACEMENT_3D('',#88260,#62310,#62311) ;
#52244=AXIS2_PLACEMENT_3D('',#88265,#62314,#62315) ;
#52245=AXIS2_PLACEMENT_3D('',#88266,#62316,#62317) ;
#52246=AXIS2_PLACEMENT_3D('',#88269,#62320,#62321) ;
#52247=AXIS2_PLACEMENT_3D('',#88274,#62324,#62325) ;
#52248=AXIS2_PLACEMENT_3D('',#88275,#62326,#62327) ;
#52249=AXIS2_PLACEMENT_3D('',#88280,#62330,#62331) ;
#52250=AXIS2_PLACEMENT_3D('',#88281,#62332,#62333) ;
#52251=AXIS2_PLACEMENT_3D('',#88286,#62336,#62337) ;
#52252=AXIS2_PLACEMENT_3D('',#88287,#62338,#62339) ;
#52253=AXIS2_PLACEMENT_3D('',#88290,#62342,#62343) ;
#52254=AXIS2_PLACEMENT_3D('',#88296,#62347,#62348) ;
#52255=AXIS2_PLACEMENT_3D('',#88300,#62351,#62352) ;
#52256=AXIS2_PLACEMENT_3D('',#88304,#62355,#62356) ;
#52257=AXIS2_PLACEMENT_3D('',#88308,#62359,#62360) ;
#52258=AXIS2_PLACEMENT_3D('',#88312,#62363,#62364) ;
#52259=AXIS2_PLACEMENT_3D('',#88316,#62367,#62368) ;
#52260=AXIS2_PLACEMENT_3D('',#88318,#62369,#62370) ;
#52261=AXIS2_PLACEMENT_3D('',#88319,#62371,#62372) ;
#52262=AXIS2_PLACEMENT_3D('',#88324,#62374,#62375) ;
#52263=AXIS2_PLACEMENT_3D('',#88327,#62377,#62378) ;
#52264=AXIS2_PLACEMENT_3D('',#88328,#62379,#62380) ;
#52265=AXIS2_PLACEMENT_3D('',#88332,#62382,#62383) ;
#52266=AXIS2_PLACEMENT_3D('',#88334,#62385,#62386) ;
#52267=AXIS2_PLACEMENT_3D('',#88338,#62388,#62389) ;
#52268=AXIS2_PLACEMENT_3D('',#88340,#62391,#62392) ;
#52269=AXIS2_PLACEMENT_3D('',#88343,#62394,#62395) ;
#52270=AXIS2_PLACEMENT_3D('',#88345,#62397,#62398) ;
#52271=AXIS2_PLACEMENT_3D('',#88348,#62400,#62401) ;
#52272=AXIS2_PLACEMENT_3D('',#88349,#62402,#62403) ;
#52273=AXIS2_PLACEMENT_3D('',#88352,#62405,#62406) ;
#52274=AXIS2_PLACEMENT_3D('',#88353,#62407,#62408) ;
#52275=AXIS2_PLACEMENT_3D('',#88356,#62410,#62411) ;
#52276=AXIS2_PLACEMENT_3D('',#88357,#62412,#62413) ;
#52277=AXIS2_PLACEMENT_3D('',#88360,#62415,#62416) ;
#52278=AXIS2_PLACEMENT_3D('',#88361,#62417,#62418) ;
#52279=AXIS2_PLACEMENT_3D('',#88364,#62420,#62421) ;
#52280=AXIS2_PLACEMENT_3D('',#88365,#62422,#62423) ;
#52281=AXIS2_PLACEMENT_3D('',#88368,#62425,#62426) ;
#52282=AXIS2_PLACEMENT_3D('',#88369,#62427,#62428) ;
#52283=AXIS2_PLACEMENT_3D('',#88374,#62431,#62432) ;
#52284=AXIS2_PLACEMENT_3D('',#88375,#62433,#62434) ;
#52285=AXIS2_PLACEMENT_3D('',#88378,#62437,#62438) ;
#52286=AXIS2_PLACEMENT_3D('',#88380,#62440,#62441) ;
#52287=AXIS2_PLACEMENT_3D('',#88382,#62443,#62444) ;
#52288=AXIS2_PLACEMENT_3D('',#88384,#62446,#62447) ;
#52289=AXIS2_PLACEMENT_3D('',#88385,#62448,#62449) ;
#52290=AXIS2_PLACEMENT_3D('',#88386,#62450,#62451) ;
#52291=AXIS2_PLACEMENT_3D('',#88387,#62452,#62453) ;
#52292=AXIS2_PLACEMENT_3D('',#88389,#62455,#62456) ;
#52293=AXIS2_PLACEMENT_3D('',#88391,#62458,#62459) ;
#62249=DIRECTION('axis',(0.,0.,1.)) ;
#62250=DIRECTION('refdir',(1.,0.,0.)) ;
#62251=DIRECTION('center_axis',(2.52374105052742E-18,5.60383084497445E-34,
-1.)) ;
#62252=DIRECTION('ref_axis',(-1.,0.,0.)) ;
#62253=DIRECTION('center_axis',(-2.52374105052742E-18,-5.60383084497445E-34,
1.)) ;
#62254=DIRECTION('ref_axis',(1.,-2.80191542248716E-35,2.52374105052742E-18)) ;
#62255=DIRECTION('center_axis',(0.,-1.,-5.60383084497445E-34)) ;
#62256=DIRECTION('ref_axis',(1.,0.,0.)) ;
#62257=DIRECTION('center_axis',(2.52374105052742E-18,5.60383084497445E-34,
-1.)) ;
#62258=DIRECTION('ref_axis',(1.,-2.80191542248716E-35,2.52374105052742E-18)) ;
#62259=DIRECTION('center_axis',(2.52374105052742E-18,5.60383084497445E-34,
-1.)) ;
#62260=DIRECTION('ref_axis',(1.,-2.80191542248716E-35,2.52374105052742E-18)) ;
#62261=DIRECTION('center_axis',(0.,0.,-1.)) ;
#62262=DIRECTION('ref_axis',(1.,0.,0.)) ;
#62263=DIRECTION('',(0.,0.,1.)) ;
#62264=DIRECTION('center_axis',(-2.52374105052742E-18,-5.60383084497445E-34,
1.)) ;
#62265=DIRECTION('ref_axis',(1.,5.60383084497445E-35,2.52374105052742E-18)) ;
#62266=DIRECTION('center_axis',(-2.52374105052742E-18,-5.60383084497445E-34,
1.)) ;
#62267=DIRECTION('ref_axis',(1.,5.60383084497445E-35,2.52374105052742E-18)) ;
#62268=DIRECTION('center_axis',(2.52374105052742E-18,5.60383084497445E-34,
-1.)) ;
#62269=DIRECTION('ref_axis',(1.,3.40207761657885E-68,2.52374105052742E-18)) ;
#62270=DIRECTION('center_axis',(-1.,0.,-2.52374105052742E-18)) ;
#62271=DIRECTION('ref_axis',(-1.78455441078696E-18,0.707106781186485,0.70710678118661)) ;
#62272=DIRECTION('',(1.,0.,2.52374105052742E-18)) ;
#62273=DIRECTION('center_axis',(-0.70710678118661,-0.707106781186485,0.)) ;
#62274=DIRECTION('ref_axis',(0.707106781186485,-0.70710678118661,3.56910882157392E-18)) ;
#62275=DIRECTION('',(-1.,0.,-2.52374105052742E-18)) ;
#62276=DIRECTION('center_axis',(-0.70710678118661,0.707106781186485,0.)) ;
#62277=DIRECTION('ref_axis',(-0.707106781186485,-0.70710678118661,-7.92501358220685E-34)) ;
#62278=DIRECTION('center_axis',(1.41426179436738E-51,-1.,-5.60383084497445E-34)) ;
#62279=DIRECTION('ref_axis',(-0.707106781186548,-3.96250679110377E-34,0.707106781186548)) ;
#62280=DIRECTION('',(-1.41426179436738E-51,1.,5.60383084497445E-34)) ;
#62281=DIRECTION('center_axis',(-0.70710678118661,-0.707106781186485,0.)) ;
#62282=DIRECTION('ref_axis',(-0.707106781186485,0.70710678118661,7.92501358220685E-34)) ;
#62283=DIRECTION('',(1.41426179436738E-51,-1.,-5.60383084497445E-34)) ;
#62284=DIRECTION('center_axis',(-1.,0.,-2.52374105052742E-18)) ;
#62285=DIRECTION('ref_axis',(-1.78455441078696E-18,0.707106781186485,0.70710678118661)) ;
#62286=DIRECTION('',(1.,0.,2.52374105052742E-18)) ;
#62287=DIRECTION('center_axis',(-0.70710678118661,-0.707106781186485,0.)) ;
#62288=DIRECTION('ref_axis',(0.707106781186485,-0.70710678118661,3.56910882157392E-18)) ;
#62289=DIRECTION('',(-1.,0.,-2.52374105052742E-18)) ;
#62290=DIRECTION('center_axis',(1.41426179436738E-51,-1.,-5.60383084497445E-34)) ;
#62291=DIRECTION('ref_axis',(-0.707106781186548,-3.96250679110377E-34,0.707106781186548)) ;
#62292=DIRECTION('',(-1.41426179436738E-51,1.,5.60383084497445E-34)) ;
#62293=DIRECTION('center_axis',(0.70710678118661,-0.707106781186485,0.)) ;
#62294=DIRECTION('ref_axis',(0.707106781186485,0.70710678118661,7.92501358220685E-34)) ;
#62295=DIRECTION('',(1.41426179436738E-51,-1.,-5.60383084497445E-34)) ;
#62296=DIRECTION('center_axis',(1.,0.,2.52374105052742E-18)) ;
#62297=DIRECTION('ref_axis',(-1.78455441078696E-18,-0.707106781186485,0.70710678118661)) ;
#62298=DIRECTION('',(-1.,0.,-2.52374105052742E-18)) ;
#62299=DIRECTION('center_axis',(0.70710678118661,-0.707106781186485,0.)) ;
#62300=DIRECTION('ref_axis',(-0.707106781186485,-0.70710678118661,-3.56910882157392E-18)) ;
#62301=DIRECTION('',(1.,0.,2.52374105052742E-18)) ;
#62302=DIRECTION('center_axis',(1.,0.,2.52374105052742E-18)) ;
#62303=DIRECTION('ref_axis',(-1.78455441078696E-18,-0.707106781186485,0.70710678118661)) ;
#62304=DIRECTION('',(-1.,0.,-2.52374105052742E-18)) ;
#62305=DIRECTION('center_axis',(0.70710678118661,0.707106781186485,0.)) ;
#62306=DIRECTION('ref_axis',(-0.707106781186485,0.70710678118661,-3.56910882157392E-18)) ;
#62307=DIRECTION('',(1.,0.,2.52374105052742E-18)) ;
#62308=DIRECTION('center_axis',(-0.70710678118661,0.707106781186485,0.)) ;
#62309=DIRECTION('ref_axis',(-0.707106781186485,-0.70710678118661,-3.56910882157392E-18)) ;
#62310=DIRECTION('center_axis',(-1.41426179436738E-51,1.,5.60383084497445E-34)) ;
#62311=DIRECTION('ref_axis',(0.707106781186548,-3.96250679110377E-34,0.707106781186548)) ;
#62312=DIRECTION('',(-1.41426179436738E-51,1.,5.60383084497445E-34)) ;
#62313=DIRECTION('',(1.41426179436738E-51,-1.,-5.60383084497445E-34)) ;
#62314=DIRECTION('center_axis',(0.70710678118661,0.707106781186485,0.)) ;
#62315=DIRECTION('ref_axis',(0.707106781186485,-0.70710678118661,-7.92501358220685E-34)) ;
#62316=DIRECTION('center_axis',(1.41426179436738E-51,-1.,-5.60383084497445E-34)) ;
#62317=DIRECTION('ref_axis',(-0.707106781186548,-3.96250679110377E-34,0.707106781186548)) ;
#62318=DIRECTION('',(-1.41426179436738E-51,1.,5.60383084497445E-34)) ;
#62319=DIRECTION('',(1.41426179436738E-51,-1.,-5.60383084497445E-34)) ;
#62320=DIRECTION('center_axis',(1.,0.,2.52374105052742E-18)) ;
#62321=DIRECTION('ref_axis',(-1.78455441078696E-18,-0.707106781186485,0.70710678118661)) ;
#62322=DIRECTION('',(1.,0.,2.52374105052742E-18)) ;
#62323=DIRECTION('',(-1.,0.,-2.52374105052742E-18)) ;
#62324=DIRECTION('center_axis',(0.70710678118661,0.707106781186485,0.)) ;
#62325=DIRECTION('ref_axis',(-0.707106781186485,0.70710678118661,-3.56910882157392E-18)) ;
#62326=DIRECTION('center_axis',(-1.41426179436738E-51,1.,5.60383084497445E-34)) ;
#62327=DIRECTION('ref_axis',(0.707106781186548,-3.96250679110377E-34,0.707106781186548)) ;
#62328=DIRECTION('',(-1.41426179436738E-51,1.,5.60383084497445E-34)) ;
#62329=DIRECTION('',(1.41426179436738E-51,-1.,-5.60383084497445E-34)) ;
#62330=DIRECTION('center_axis',(-0.70710678118661,0.707106781186485,0.)) ;
#62331=DIRECTION('ref_axis',(-0.707106781186485,-0.70710678118661,-7.92501358220685E-34)) ;
#62332=DIRECTION('center_axis',(-1.,0.,-2.52374105052742E-18)) ;
#62333=DIRECTION('ref_axis',(-1.78455441078696E-18,0.707106781186485,0.70710678118661)) ;
#62334=DIRECTION('',(-1.,0.,-2.52374105052742E-18)) ;
#62335=DIRECTION('',(1.,0.,2.52374105052742E-18)) ;
#62336=DIRECTION('center_axis',(-0.70710678118661,0.707106781186485,0.)) ;
#62337=DIRECTION('ref_axis',(0.707106781186485,0.70710678118661,3.56910882157392E-18)) ;
#62338=DIRECTION('center_axis',(-1.41426179436738E-51,1.,5.60383084497445E-34)) ;
#62339=DIRECTION('ref_axis',(0.707106781186548,-3.96250679110377E-34,0.707106781186548)) ;
#62340=DIRECTION('',(-1.41426179436738E-51,1.,5.60383084497445E-34)) ;
#62341=DIRECTION('',(1.41426179436738E-51,-1.,-5.60383084497445E-34)) ;
#62342=DIRECTION('center_axis',(1.,1.41426179436738E-51,0.)) ;
#62343=DIRECTION('ref_axis',(1.41426179436738E-51,-1.,-5.60383084497445E-34)) ;
#62344=DIRECTION('',(0.,0.,-1.)) ;
#62345=DIRECTION('',(-1.41426179436738E-51,1.,0.)) ;
#62346=DIRECTION('',(0.,0.,-1.)) ;
#62347=DIRECTION('center_axis',(0.,-1.,0.)) ;
#62348=DIRECTION('ref_axis',(-1.,0.,-2.52374105052742E-18)) ;
#62349=DIRECTION('',(0.,0.,-1.)) ;
#62350=DIRECTION('',(1.,0.,0.)) ;
#62351=DIRECTION('center_axis',(1.,1.41426179436738E-51,0.)) ;
#62352=DIRECTION('ref_axis',(1.41426179436738E-51,-1.,-5.60383084497445E-34)) ;
#62353=DIRECTION('',(0.,0.,-1.)) ;
#62354=DIRECTION('',(-1.41426179436738E-51,1.,0.)) ;
#62355=DIRECTION('center_axis',(0.,1.,0.)) ;
#62356=DIRECTION('ref_axis',(1.,0.,2.52374105052742E-18)) ;
#62357=DIRECTION('',(0.,0.,-1.)) ;
#62358=DIRECTION('',(-1.,0.,0.)) ;
#62359=DIRECTION('center_axis',(1.,1.41426179436738E-51,0.)) ;
#62360=DIRECTION('ref_axis',(1.41426179436738E-51,-1.,-5.60383084497445E-34)) ;
#62361=DIRECTION('',(0.,0.,-1.)) ;
#62362=DIRECTION('',(-1.41426179436738E-51,1.,0.)) ;
#62363=DIRECTION('center_axis',(0.,1.,0.)) ;
#62364=DIRECTION('ref_axis',(1.,0.,2.52374105052742E-18)) ;
#62365=DIRECTION('',(0.,0.,-1.)) ;
#62366=DIRECTION('',(-1.,0.,0.)) ;
#62367=DIRECTION('center_axis',(2.52374105052742E-18,5.60383084497445E-34,
-1.)) ;
#62368=DIRECTION('ref_axis',(1.,3.40207761657885E-68,2.52374105052742E-18)) ;
#62369=DIRECTION('center_axis',(2.52374105052742E-18,5.60383084497445E-34,
-1.)) ;
#62370=DIRECTION('ref_axis',(1.,5.60383084497445E-35,2.52374105052742E-18)) ;
#62371=DIRECTION('center_axis',(-1.,0.,0.)) ;
#62372=DIRECTION('ref_axis',(0.,-0.707106781186736,-0.707106781186359)) ;
#62373=DIRECTION('',(-1.,0.,0.)) ;
#62374=DIRECTION('center_axis',(-0.707106781186736,0.707106781186359,0.)) ;
#62375=DIRECTION('ref_axis',(0.707106781186359,0.707106781186736,0.)) ;
#62376=DIRECTION('',(1.,0.,0.)) ;
#62377=DIRECTION('center_axis',(-0.707106781186736,0.707106781186359,0.)) ;
#62378=DIRECTION('ref_axis',(-0.707106781186359,-0.707106781186736,0.)) ;
#62379=DIRECTION('center_axis',(-1.41426179436738E-51,1.,0.)) ;
#62380=DIRECTION('ref_axis',(-0.707106781186548,-1.00003410517023E-51,-0.707106781186548)) ;
#62381=DIRECTION('',(-1.41426179436738E-51,1.,0.)) ;
#62382=DIRECTION('center_axis',(0.707106781186736,0.707106781186359,0.)) ;
#62383=DIRECTION('ref_axis',(0.707106781186359,-0.707106781186736,0.)) ;
#62384=DIRECTION('',(1.41426179436738E-51,-1.,0.)) ;
#62385=DIRECTION('center_axis',(1.,0.,0.)) ;
#62386=DIRECTION('ref_axis',(0.,0.707106781186736,-0.707106781186359)) ;
#62387=DIRECTION('',(1.,0.,0.)) ;
#62388=DIRECTION('center_axis',(0.707106781186736,0.707106781186359,0.)) ;
#62389=DIRECTION('ref_axis',(-0.707106781186359,0.707106781186736,0.)) ;
#62390=DIRECTION('',(-1.,0.,0.)) ;
#62391=DIRECTION('center_axis',(-1.41426179436738E-51,1.,0.)) ;
#62392=DIRECTION('ref_axis',(-0.707106781186548,-1.00003410517023E-51,-0.707106781186548)) ;
#62393=DIRECTION('',(-1.41426179436738E-51,1.,0.)) ;
#62394=DIRECTION('center_axis',(0.707106781186485,0.70710678118661,0.)) ;
#62395=DIRECTION('ref_axis',(0.70710678118661,-0.707106781186485,0.)) ;
#62396=DIRECTION('',(1.41426179436738E-51,-1.,0.)) ;
#62397=DIRECTION('center_axis',(1.,0.,0.)) ;
#62398=DIRECTION('ref_axis',(0.,0.707106781186485,-0.70710678118661)) ;
#62399=DIRECTION('',(1.,0.,0.)) ;
#62400=DIRECTION('center_axis',(0.707106781186485,-0.70710678118661,0.)) ;
#62401=DIRECTION('ref_axis',(-0.70710678118661,-0.707106781186485,0.)) ;
#62402=DIRECTION('center_axis',(1.41426179436738E-51,-1.,0.)) ;
#62403=DIRECTION('ref_axis',(0.707106781186548,1.00003410517023E-51,-0.707106781186548)) ;
#62404=DIRECTION('',(1.41426179436738E-51,-1.,0.)) ;
#62405=DIRECTION('center_axis',(0.707106781186736,-0.707106781186359,0.)) ;
#62406=DIRECTION('ref_axis',(0.707106781186359,0.707106781186736,0.)) ;
#62407=DIRECTION('center_axis',(1.,0.,0.)) ;
#62408=DIRECTION('ref_axis',(0.,0.707106781186736,-0.707106781186359)) ;
#62409=DIRECTION('',(1.,0.,0.)) ;
#62410=DIRECTION('center_axis',(0.707106781186736,-0.707106781186359,0.)) ;
#62411=DIRECTION('ref_axis',(-0.707106781186359,-0.707106781186736,0.)) ;
#62412=DIRECTION('center_axis',(1.41426179436738E-51,-1.,0.)) ;
#62413=DIRECTION('ref_axis',(0.707106781186548,1.00003410517023E-51,-0.707106781186548)) ;
#62414=DIRECTION('',(1.41426179436738E-51,-1.,0.)) ;
#62415=DIRECTION('center_axis',(-0.707106781186736,-0.707106781186359,0.)) ;
#62416=DIRECTION('ref_axis',(-0.707106781186359,0.707106781186736,0.)) ;
#62417=DIRECTION('center_axis',(-1.,0.,0.)) ;
#62418=DIRECTION('ref_axis',(0.,-0.707106781186736,-0.707106781186359)) ;
#62419=DIRECTION('',(-1.,0.,0.)) ;
#62420=DIRECTION('center_axis',(-0.707106781186736,-0.707106781186359,0.)) ;
#62421=DIRECTION('ref_axis',(0.707106781186359,-0.707106781186736,0.)) ;
#62422=DIRECTION('center_axis',(1.41426179436738E-51,-1.,0.)) ;
#62423=DIRECTION('ref_axis',(0.707106781186548,1.00003410517023E-51,-0.707106781186548)) ;
#62424=DIRECTION('',(1.41426179436738E-51,-1.,0.)) ;
#62425=DIRECTION('center_axis',(-0.707106781186485,-0.70710678118661,0.)) ;
#62426=DIRECTION('ref_axis',(-0.70710678118661,0.707106781186485,0.)) ;
#62427=DIRECTION('center_axis',(-1.,0.,0.)) ;
#62428=DIRECTION('ref_axis',(0.,-0.707106781186485,-0.70710678118661)) ;
#62429=DIRECTION('',(1.,0.,0.)) ;
#62430=DIRECTION('',(-1.,0.,0.)) ;
#62431=DIRECTION('center_axis',(-0.707106781186485,0.70710678118661,0.)) ;
#62432=DIRECTION('ref_axis',(0.70710678118661,0.707106781186485,0.)) ;
#62433=DIRECTION('center_axis',(-1.41426179436738E-51,1.,0.)) ;
#62434=DIRECTION('ref_axis',(-0.707106781186548,-1.00003410517023E-51,-0.707106781186548)) ;
#62435=DIRECTION('',(1.41426179436738E-51,-1.,0.)) ;
#62436=DIRECTION('',(-1.41426179436738E-51,1.,0.)) ;
#62437=DIRECTION('center_axis',(0.,-1.,0.)) ;
#62438=DIRECTION('ref_axis',(-1.,0.,-2.52374105052742E-18)) ;
#62439=DIRECTION('',(0.,0.,-1.)) ;
#62440=DIRECTION('center_axis',(-1.,-1.41426179436738E-51,0.)) ;
#62441=DIRECTION('ref_axis',(-1.41426179436738E-51,1.,5.60383084497445E-34)) ;
#62442=DIRECTION('',(0.,0.,-1.)) ;
#62443=DIRECTION('center_axis',(0.,-1.,0.)) ;
#62444=DIRECTION('ref_axis',(-1.,0.,-2.52374105052742E-18)) ;
#62445=DIRECTION('',(0.,0.,-1.)) ;
#62446=DIRECTION('center_axis',(0.,0.,-1.)) ;
#62447=DIRECTION('ref_axis',(-1.,0.,0.)) ;
#62448=DIRECTION('center_axis',(2.52374105052742E-18,5.60383084497445E-34,
-1.)) ;
#62449=DIRECTION('ref_axis',(-1.,0.,0.)) ;
#62450=DIRECTION('center_axis',(0.,-1.,-5.60383084497445E-34)) ;
#62451=DIRECTION('ref_axis',(1.,0.,0.)) ;
#62452=DIRECTION('center_axis',(-1.,-1.41426179436738E-51,0.)) ;
#62453=DIRECTION('ref_axis',(-1.41426179436738E-51,1.,5.60383084497445E-34)) ;
#62454=DIRECTION('',(0.,0.,-1.)) ;
#62455=DIRECTION('center_axis',(0.,1.,0.)) ;
#62456=DIRECTION('ref_axis',(1.,0.,2.52374105052742E-18)) ;
#62457=DIRECTION('',(0.,0.,-1.)) ;
#62458=DIRECTION('center_axis',(-1.,-1.41426179436738E-51,0.)) ;
#62459=DIRECTION('ref_axis',(-1.41426179436738E-51,1.,5.60383084497445E-34)) ;
#88202=CARTESIAN_POINT('',(0.,0.,0.)) ;
#88203=CARTESIAN_POINT('Origin',(64.1568347953872,220.146231446812,28.8213203435596)) ;
#88204=CARTESIAN_POINT('',(66.0568347953872,220.146231446812,28.7213203435596)) ;
#88205=CARTESIAN_POINT('Origin',(64.1568347953872,220.146231446812,28.7213203435596)) ;
#88206=CARTESIAN_POINT('',(66.1568347953872,220.146231446812,28.8213203435596)) ;
#88207=CARTESIAN_POINT('Origin',(66.0568347953872,220.146231446812,28.8213203435596)) ;
#88208=CARTESIAN_POINT('',(62.1568347953872,220.146231446812,28.8213203435596)) ;
#88209=CARTESIAN_POINT('Origin',(64.1568347953872,220.146231446812,28.8213203435596)) ;
#88210=CARTESIAN_POINT('Origin',(64.1568347953872,220.146231446812,28.8213203435596)) ;
#88211=CARTESIAN_POINT('Origin',(64.1568347953872,220.146231446812,30.2213203435596)) ;
#88212=CARTESIAN_POINT('',(62.1568347953872,220.146231446812,30.0213203435596)) ;
#88213=CARTESIAN_POINT('',(62.1568347953872,220.146231446812,30.2213203435596)) ;
#88214=CARTESIAN_POINT('',(66.1568347953872,220.146231446812,30.0213203435596)) ;
#88215=CARTESIAN_POINT('Origin',(64.1568347953872,220.146231446812,30.0213203435596)) ;
#88216=CARTESIAN_POINT('Origin',(64.1568347953872,220.146231446812,30.0213203435596)) ;
#88217=CARTESIAN_POINT('Origin',(64.1568347953872,220.146231446812,28.7213203435596)) ;
#88218=CARTESIAN_POINT('Origin',(64.3068347953872,218.546231446812,30.1213203435596)) ;
#88219=CARTESIAN_POINT('',(63.7568347953872,218.546231446812,30.2213203435596)) ;
#88220=CARTESIAN_POINT('',(64.5568347953872,218.546231446812,30.2213203435596)) ;
#88221=CARTESIAN_POINT('',(64.3068347953872,218.546231446812,30.2213203435596)) ;
#88222=CARTESIAN_POINT('',(64.4568347953872,218.646231446812,30.1213203435596)) ;
#88223=CARTESIAN_POINT('Origin',(64.5568347953872,218.546231446812,30.1213203435596)) ;
#88224=CARTESIAN_POINT('',(63.8568347953872,218.646231446812,30.1213203435596)) ;
#88225=CARTESIAN_POINT('',(64.3068347953872,218.646231446812,30.1213203435596)) ;
#88226=CARTESIAN_POINT('Origin',(63.7568347953872,218.546231446812,30.1213203435596)) ;
#88227=CARTESIAN_POINT('Origin',(64.5568347953872,219.996231446812,30.1213203435596)) ;
#88228=CARTESIAN_POINT('',(64.5568347953872,219.746231446812,30.2213203435596)) ;
#88229=CARTESIAN_POINT('',(64.5568347953872,219.996231446812,30.2213203435596)) ;
#88230=CARTESIAN_POINT('',(64.4568347953872,219.846231446812,30.1213203435596)) ;
#88231=CARTESIAN_POINT('Origin',(64.5568347953872,219.746231446812,30.1213203435596)) ;
#88232=CARTESIAN_POINT('',(64.4568347953872,219.996231446812,30.1213203435596)) ;
#88233=CARTESIAN_POINT('Origin',(64.9068347953872,219.746231446812,30.1213203435596)) ;
#88234=CARTESIAN_POINT('',(65.7568347953872,219.746231446812,30.2213203435596)) ;
#88235=CARTESIAN_POINT('',(64.9068347953872,219.746231446812,30.2213203435596)) ;
#88236=CARTESIAN_POINT('',(65.6568347953872,219.846231446812,30.1213203435596)) ;
#88237=CARTESIAN_POINT('Origin',(65.7568347953872,219.746231446812,30.1213203435596)) ;
#88238=CARTESIAN_POINT('',(64.9068347953872,219.846231446812,30.1213203435596)) ;
#88239=CARTESIAN_POINT('Origin',(65.7568347953872,220.296231446812,30.1213203435596)) ;
#88240=CARTESIAN_POINT('',(65.7568347953872,220.546231446812,30.2213203435596)) ;
#88241=CARTESIAN_POINT('',(65.7568347953872,220.296231446812,30.2213203435596)) ;
#88242=CARTESIAN_POINT('',(65.6568347953872,220.446231446812,30.1213203435596)) ;
#88243=CARTESIAN_POINT('Origin',(65.7568347953872,220.546231446812,30.1213203435596)) ;
#88244=CARTESIAN_POINT('',(65.6568347953872,220.296231446812,30.1213203435596)) ;
#88245=CARTESIAN_POINT('Origin',(64.3068347953872,220.546231446812,30.1213203435596)) ;
#88246=CARTESIAN_POINT('',(64.5568347953872,220.546231446812,30.2213203435596)) ;
#88247=CARTESIAN_POINT('',(64.3068347953872,220.546231446812,30.2213203435596)) ;
#88248=CARTESIAN_POINT('',(64.4568347953872,220.446231446812,30.1213203435596)) ;
#88249=CARTESIAN_POINT('Origin',(64.5568347953872,220.546231446812,30.1213203435596)) ;
#88250=CARTESIAN_POINT('',(64.3068347953872,220.446231446812,30.1213203435596)) ;
#88251=CARTESIAN_POINT('Origin',(64.0068347953872,221.746231446812,30.1213203435596)) ;
#88252=CARTESIAN_POINT('',(64.5568347953872,221.746231446812,30.2213203435596)) ;
#88253=CARTESIAN_POINT('',(63.7568347953872,221.746231446812,30.2213203435596)) ;
#88254=CARTESIAN_POINT('',(64.0068347953872,221.746231446812,30.2213203435596)) ;
#88255=CARTESIAN_POINT('',(63.8568347953872,221.646231446812,30.1213203435596)) ;
#88256=CARTESIAN_POINT('Origin',(63.7568347953872,221.746231446812,30.1213203435596)) ;
#88257=CARTESIAN_POINT('',(64.4568347953872,221.646231446812,30.1213203435596)) ;
#88258=CARTESIAN_POINT('',(64.0068347953872,221.646231446812,30.1213203435596)) ;
#88259=CARTESIAN_POINT('Origin',(64.5568347953872,221.746231446812,30.1213203435596)) ;
#88260=CARTESIAN_POINT('Origin',(63.7568347953872,220.296231446812,30.1213203435596)) ;
#88261=CARTESIAN_POINT('',(63.8568347953872,220.446231446812,30.1213203435596)) ;
#88262=CARTESIAN_POINT('',(63.8568347953872,220.296231446812,30.1213203435596)) ;
#88263=CARTESIAN_POINT('',(63.7568347953872,220.546231446812,30.2213203435596)) ;
#88264=CARTESIAN_POINT('',(63.7568347953872,220.296231446812,30.2213203435596)) ;
#88265=CARTESIAN_POINT('Origin',(63.7568347953872,220.546231446812,30.1213203435596)) ;
#88266=CARTESIAN_POINT('Origin',(64.5568347953872,220.896231446812,30.1213203435596)) ;
#88267=CARTESIAN_POINT('',(64.5568347953872,220.896231446812,30.2213203435596)) ;
#88268=CARTESIAN_POINT('',(64.4568347953872,220.896231446812,30.1213203435596)) ;
#88269=CARTESIAN_POINT('Origin',(63.4068347953872,220.546231446812,30.1213203435596)) ;
#88270=CARTESIAN_POINT('',(62.6568347953872,220.446231446812,30.1213203435596)) ;
#88271=CARTESIAN_POINT('',(63.4068347953872,220.446231446812,30.1213203435596)) ;
#88272=CARTESIAN_POINT('',(62.5568347953872,220.546231446812,30.2213203435596)) ;
#88273=CARTESIAN_POINT('',(63.4068347953872,220.546231446812,30.2213203435596)) ;
#88274=CARTESIAN_POINT('Origin',(62.5568347953872,220.546231446812,30.1213203435596)) ;
#88275=CARTESIAN_POINT('Origin',(62.5568347953872,219.996231446812,30.1213203435596)) ;
#88276=CARTESIAN_POINT('',(62.6568347953872,219.846231446812,30.1213203435596)) ;
#88277=CARTESIAN_POINT('',(62.6568347953872,219.996231446812,30.1213203435596)) ;
#88278=CARTESIAN_POINT('',(62.5568347953872,219.746231446812,30.2213203435596)) ;
#88279=CARTESIAN_POINT('',(62.5568347953872,219.996231446812,30.2213203435596)) ;
#88280=CARTESIAN_POINT('Origin',(62.5568347953872,219.746231446812,30.1213203435596)) ;
#88281=CARTESIAN_POINT('Origin',(64.0068347953872,219.746231446812,30.1213203435596)) ;
#88282=CARTESIAN_POINT('',(63.8568347953872,219.846231446812,30.1213203435596)) ;
#88283=CARTESIAN_POINT('',(64.0068347953872,219.846231446812,30.1213203435596)) ;
#88284=CARTESIAN_POINT('',(63.7568347953872,219.746231446812,30.2213203435596)) ;
#88285=CARTESIAN_POINT('',(64.0068347953872,219.746231446812,30.2213203435596)) ;
#88286=CARTESIAN_POINT('Origin',(63.7568347953872,219.746231446812,30.1213203435596)) ;
#88287=CARTESIAN_POINT('Origin',(63.7568347953872,219.396231446812,30.1213203435596)) ;
#88288=CARTESIAN_POINT('',(63.8568347953872,219.396231446812,30.1213203435596)) ;
#88289=CARTESIAN_POINT('',(63.7568347953872,219.396231446812,30.2213203435596)) ;
#88290=CARTESIAN_POINT('Origin',(64.4568347953872,219.846231446812,30.7213203435596)) ;
#88291=CARTESIAN_POINT('',(64.4568347953872,219.846231446812,30.0213203435596)) ;
#88292=CARTESIAN_POINT('',(64.4568347953872,219.846231446812,30.7213203435596)) ;
#88293=CARTESIAN_POINT('',(64.4568347953872,218.646231446812,30.0213203435596)) ;
#88294=CARTESIAN_POINT('',(64.4568347953872,219.996231446812,30.0213203435596)) ;
#88295=CARTESIAN_POINT('',(64.4568347953872,218.646231446812,30.7213203435596)) ;
#88296=CARTESIAN_POINT('Origin',(65.6568347953872,219.846231446812,30.7213203435596)) ;
#88297=CARTESIAN_POINT('',(65.6568347953872,219.846231446812,30.0213203435596)) ;
#88298=CARTESIAN_POINT('',(65.6568347953872,219.846231446812,30.7213203435596)) ;
#88299=CARTESIAN_POINT('',(64.9068347953872,219.846231446812,30.0213203435596)) ;
#88300=CARTESIAN_POINT('Origin',(65.6568347953872,220.446231446812,30.7213203435596)) ;
#88301=CARTESIAN_POINT('',(65.6568347953872,220.446231446812,30.0213203435596)) ;
#88302=CARTESIAN_POINT('',(65.6568347953872,220.446231446812,30.7213203435596)) ;
#88303=CARTESIAN_POINT('',(65.6568347953872,220.296231446812,30.0213203435596)) ;
#88304=CARTESIAN_POINT('Origin',(64.4568347953872,220.446231446812,30.7213203435596)) ;
#88305=CARTESIAN_POINT('',(64.4568347953872,220.446231446812,30.0213203435596)) ;
#88306=CARTESIAN_POINT('',(64.4568347953872,220.446231446812,30.7213203435596)) ;
#88307=CARTESIAN_POINT('',(64.3068347953872,220.446231446812,30.0213203435596)) ;
#88308=CARTESIAN_POINT('Origin',(64.4568347953872,221.646231446812,30.7213203435596)) ;
#88309=CARTESIAN_POINT('',(64.4568347953872,221.646231446812,30.0213203435596)) ;
#88310=CARTESIAN_POINT('',(64.4568347953872,221.646231446812,30.7213203435596)) ;
#88311=CARTESIAN_POINT('',(64.4568347953872,220.896231446812,30.0213203435596)) ;
#88312=CARTESIAN_POINT('Origin',(63.8568347953872,221.646231446812,30.7213203435596)) ;
#88313=CARTESIAN_POINT('',(63.8568347953872,221.646231446812,30.0213203435596)) ;
#88314=CARTESIAN_POINT('',(63.8568347953872,221.646231446812,30.7213203435596)) ;
#88315=CARTESIAN_POINT('',(64.0068347953872,221.646231446812,30.0213203435596)) ;
#88316=CARTESIAN_POINT('Origin',(64.1568347953872,220.146231446812,30.2213203435596)) ;
#88317=CARTESIAN_POINT('',(65.9568347953872,220.146231446812,30.2213203435596)) ;
#88318=CARTESIAN_POINT('Origin',(64.1568347953872,220.146231446812,30.2213203435596)) ;
#88319=CARTESIAN_POINT('Origin',(64.0068347953872,219.946231446812,30.0213203435596)) ;
#88320=CARTESIAN_POINT('',(63.9568347953872,219.946231446812,29.9213203435596)) ;
#88321=CARTESIAN_POINT('',(62.7568347953872,219.946231446812,29.9213203435596)) ;
#88322=CARTESIAN_POINT('',(64.0068347953872,219.946231446812,29.9213203435596)) ;
#88323=CARTESIAN_POINT('',(62.6568347953872,219.846231446812,30.0213203435596)) ;
#88324=CARTESIAN_POINT('Origin',(62.7568347953872,219.946231446812,30.0213203435596)) ;
#88325=CARTESIAN_POINT('',(63.8568347953872,219.846231446812,30.0213203435596)) ;
#88326=CARTESIAN_POINT('',(64.0068347953872,219.846231446812,30.0213203435596)) ;
#88327=CARTESIAN_POINT('Origin',(63.9568347953872,219.946231446812,30.0213203435596)) ;
#88328=CARTESIAN_POINT('Origin',(62.7568347953872,219.996231446812,30.0213203435596)) ;
#88329=CARTESIAN_POINT('',(62.7568347953872,220.346231446812,29.9213203435596)) ;
#88330=CARTESIAN_POINT('',(62.7568347953872,219.996231446812,29.9213203435596)) ;
#88331=CARTESIAN_POINT('',(62.6568347953872,220.446231446812,30.0213203435596)) ;
#88332=CARTESIAN_POINT('Origin',(62.7568347953872,220.346231446812,30.0213203435596)) ;
#88333=CARTESIAN_POINT('',(62.6568347953872,219.996231446812,30.0213203435596)) ;
#88334=CARTESIAN_POINT('Origin',(63.4068347953872,220.346231446812,30.0213203435596)) ;
#88335=CARTESIAN_POINT('',(63.9568347953872,220.346231446812,29.9213203435596)) ;
#88336=CARTESIAN_POINT('',(63.4068347953872,220.346231446812,29.9213203435596)) ;
#88337=CARTESIAN_POINT('',(63.8568347953872,220.446231446812,30.0213203435596)) ;
#88338=CARTESIAN_POINT('Origin',(63.9568347953872,220.346231446812,30.0213203435596)) ;
#88339=CARTESIAN_POINT('',(63.4068347953872,220.446231446812,30.0213203435596)) ;
#88340=CARTESIAN_POINT('Origin',(63.9568347953872,220.296231446812,30.0213203435596)) ;
#88341=CARTESIAN_POINT('',(63.9568347953872,221.546231446812,29.9213203435596)) ;
#88342=CARTESIAN_POINT('',(63.9568347953872,220.296231446812,29.9213203435596)) ;
#88343=CARTESIAN_POINT('Origin',(63.9568347953872,221.546231446812,30.0213203435596)) ;
#88344=CARTESIAN_POINT('',(63.8568347953872,220.296231446812,30.0213203435596)) ;
#88345=CARTESIAN_POINT('Origin',(64.0068347953872,221.546231446812,30.0213203435596)) ;
#88346=CARTESIAN_POINT('',(64.3568347953872,221.546231446812,29.9213203435596)) ;
#88347=CARTESIAN_POINT('',(64.0068347953872,221.546231446812,29.9213203435596)) ;
#88348=CARTESIAN_POINT('Origin',(64.3568347953872,221.546231446812,30.0213203435596)) ;
#88349=CARTESIAN_POINT('Origin',(64.3568347953872,220.896231446812,30.0213203435596)) ;
#88350=CARTESIAN_POINT('',(64.3568347953872,220.346231446812,29.9213203435596)) ;
#88351=CARTESIAN_POINT('',(64.3568347953872,220.896231446812,29.9213203435596)) ;
#88352=CARTESIAN_POINT('Origin',(64.3568347953872,220.346231446812,30.0213203435596)) ;
#88353=CARTESIAN_POINT('Origin',(64.3068347953872,220.346231446812,30.0213203435596)) ;
#88354=CARTESIAN_POINT('',(65.5568347953872,220.346231446812,29.9213203435596)) ;
#88355=CARTESIAN_POINT('',(64.3068347953872,220.346231446812,29.9213203435596)) ;
#88356=CARTESIAN_POINT('Origin',(65.5568347953872,220.346231446812,30.0213203435596)) ;
#88357=CARTESIAN_POINT('Origin',(65.5568347953872,220.296231446812,30.0213203435596)) ;
#88358=CARTESIAN_POINT('',(65.5568347953872,219.946231446812,29.9213203435596)) ;
#88359=CARTESIAN_POINT('',(65.5568347953872,220.296231446812,29.9213203435596)) ;
#88360=CARTESIAN_POINT('Origin',(65.5568347953872,219.946231446812,30.0213203435596)) ;
#88361=CARTESIAN_POINT('Origin',(64.9068347953872,219.946231446812,30.0213203435596)) ;
#88362=CARTESIAN_POINT('',(64.3568347953872,219.946231446812,29.9213203435596)) ;
#88363=CARTESIAN_POINT('',(64.9068347953872,219.946231446812,29.9213203435596)) ;
#88364=CARTESIAN_POINT('Origin',(64.3568347953872,219.946231446812,30.0213203435596)) ;
#88365=CARTESIAN_POINT('Origin',(64.3568347953872,219.996231446812,30.0213203435596)) ;
#88366=CARTESIAN_POINT('',(64.3568347953872,218.746231446812,29.9213203435596)) ;
#88367=CARTESIAN_POINT('',(64.3568347953872,219.996231446812,29.9213203435596)) ;
#88368=CARTESIAN_POINT('Origin',(64.3568347953872,218.746231446812,30.0213203435596)) ;
#88369=CARTESIAN_POINT('Origin',(64.3068347953872,218.746231446812,30.0213203435596)) ;
#88370=CARTESIAN_POINT('',(63.8568347953872,218.646231446812,30.0213203435596)) ;
#88371=CARTESIAN_POINT('',(64.3068347953872,218.646231446812,30.0213203435596)) ;
#88372=CARTESIAN_POINT('',(63.9568347953872,218.746231446812,29.9213203435596)) ;
#88373=CARTESIAN_POINT('',(64.3068347953872,218.746231446812,29.9213203435596)) ;
#88374=CARTESIAN_POINT('Origin',(63.9568347953872,218.746231446812,30.0213203435596)) ;
#88375=CARTESIAN_POINT('Origin',(63.9568347953872,219.396231446812,30.0213203435596)) ;
#88376=CARTESIAN_POINT('',(63.8568347953872,219.396231446812,30.0213203435596)) ;
#88377=CARTESIAN_POINT('',(63.9568347953872,219.396231446812,29.9213203435596)) ;
#88378=CARTESIAN_POINT('Origin',(64.4568347953872,218.646231446812,30.7213203435596)) ;
#88379=CARTESIAN_POINT('',(63.8568347953872,218.646231446812,30.7213203435596)) ;
#88380=CARTESIAN_POINT('Origin',(63.8568347953872,218.646231446812,30.7213203435596)) ;
#88381=CARTESIAN_POINT('',(63.8568347953872,219.846231446812,30.7213203435596)) ;
#88382=CARTESIAN_POINT('Origin',(63.8568347953872,219.846231446812,30.7213203435596)) ;
#88383=CARTESIAN_POINT('',(62.6568347953872,219.846231446812,30.7213203435596)) ;
#88384=CARTESIAN_POINT('Origin',(64.1568347953872,220.146231446812,29.9213203435596)) ;
#88385=CARTESIAN_POINT('Origin',(64.1568347953872,220.146231446812,30.0213203435596)) ;
#88386=CARTESIAN_POINT('Origin',(65.9568347953872,220.146231446812,30.0213203435596)) ;
#88387=CARTESIAN_POINT('Origin',(62.6568347953872,219.846231446812,30.7213203435596)) ;
#88388=CARTESIAN_POINT('',(62.6568347953872,220.446231446812,30.7213203435596)) ;
#88389=CARTESIAN_POINT('Origin',(62.6568347953872,220.446231446812,30.7213203435596)) ;
#88390=CARTESIAN_POINT('',(63.8568347953872,220.446231446812,30.7213203435596)) ;
#88391=CARTESIAN_POINT('Origin',(63.8568347953872,220.446231446812,30.7213203435596)) ;
#117137=UNCERTAINTY_MEASURE_WITH_UNIT(LENGTH_MEASURE(0.01),#117171,
'DISTANCE_ACCURACY_VALUE',
'Maximum model space distance between geometric entities at asserted c
onnectivities') ;
#117147=UNCERTAINTY_MEASURE_WITH_UNIT(LENGTH_MEASURE(0.01),#117171,
'DISTANCE_ACCURACY_VALUE',
'Maximum model space distance between geometric entities at asserted c
onnectivities') ;
#117160=(
GEOMETRIC_REPRESENTATION_CONTEXT(3)
GLOBAL_UNCERTAINTY_ASSIGNED_CONTEXT((#117137))
GLOBAL_UNIT_ASSIGNED_CONTEXT((#117171,#117173,#117174))
REPRESENTATION_CONTEXT('','3D')
) ;
#117170=(
GEOMETRIC_REPRESENTATION_CONTEXT(3)
GLOBAL_UNCERTAINTY_ASSIGNED_CONTEXT((#117147))
GLOBAL_UNIT_ASSIGNED_CONTEXT((#117171,#117173,#117174))
REPRESENTATION_CONTEXT('','3D')
) ;
#117171=(
LENGTH_UNIT()
NAMED_UNIT(*)
SI_UNIT(.MILLI.,.METRE.)
) ;
#117173=(
NAMED_UNIT(*)
PLANE_ANGLE_UNIT()
SI_UNIT($,.RADIAN.)
) ;
#117174=(
NAMED_UNIT(*)
SI_UNIT($,.STERADIAN.)
SOLID_ANGLE_UNIT()
) ;
#117187=SHAPE_DEFINITION_REPRESENTATION(#117209,#117252) ;
#117209=PRODUCT_DEFINITION_SHAPE('',$,#117275) ;
#117252=SHAPE_REPRESENTATION('',(#52219),#117160) ;
#117262=PRODUCT_DEFINITION_CONTEXT('part definition',#117330,'design') ;
#117275=PRODUCT_DEFINITION('Spacer_1','Spacer_1',#117297,#117262) ;
#117297=PRODUCT_DEFINITION_FORMATION('',$,#117344) ;
#117330=APPLICATION_CONTEXT(
'Core Data for Automotive Mechanical Design Process') ;
#117331=PRODUCT_CONTEXT('part definition',#117330,'mechanical') ;
#117344=PRODUCT('Spacer_1','Spacer_1',$,(#117331)) ;
#117355=PRESENTATION_STYLE_ASSIGNMENT((#117357)) ;
#117357=SURFACE_STYLE_USAGE(.BOTH.,#117359) ;
#117359=SURFACE_SIDE_STYLE('',(#117361)) ;
#117361=SURFACE_STYLE_FILL_AREA(#117363) ;
#117363=FILL_AREA_STYLE('Opaque(160,160,160)',(#117365)) ;
#117365=FILL_AREA_STYLE_COLOUR('Opaque(160,160,160)',#117367) ;
#117367=COLOUR_RGB('Opaque(160,160,160)', 0.09019608, 0.27058824, 0.51372549) ;
ENDSEC;
END-ISO-10303-21;
